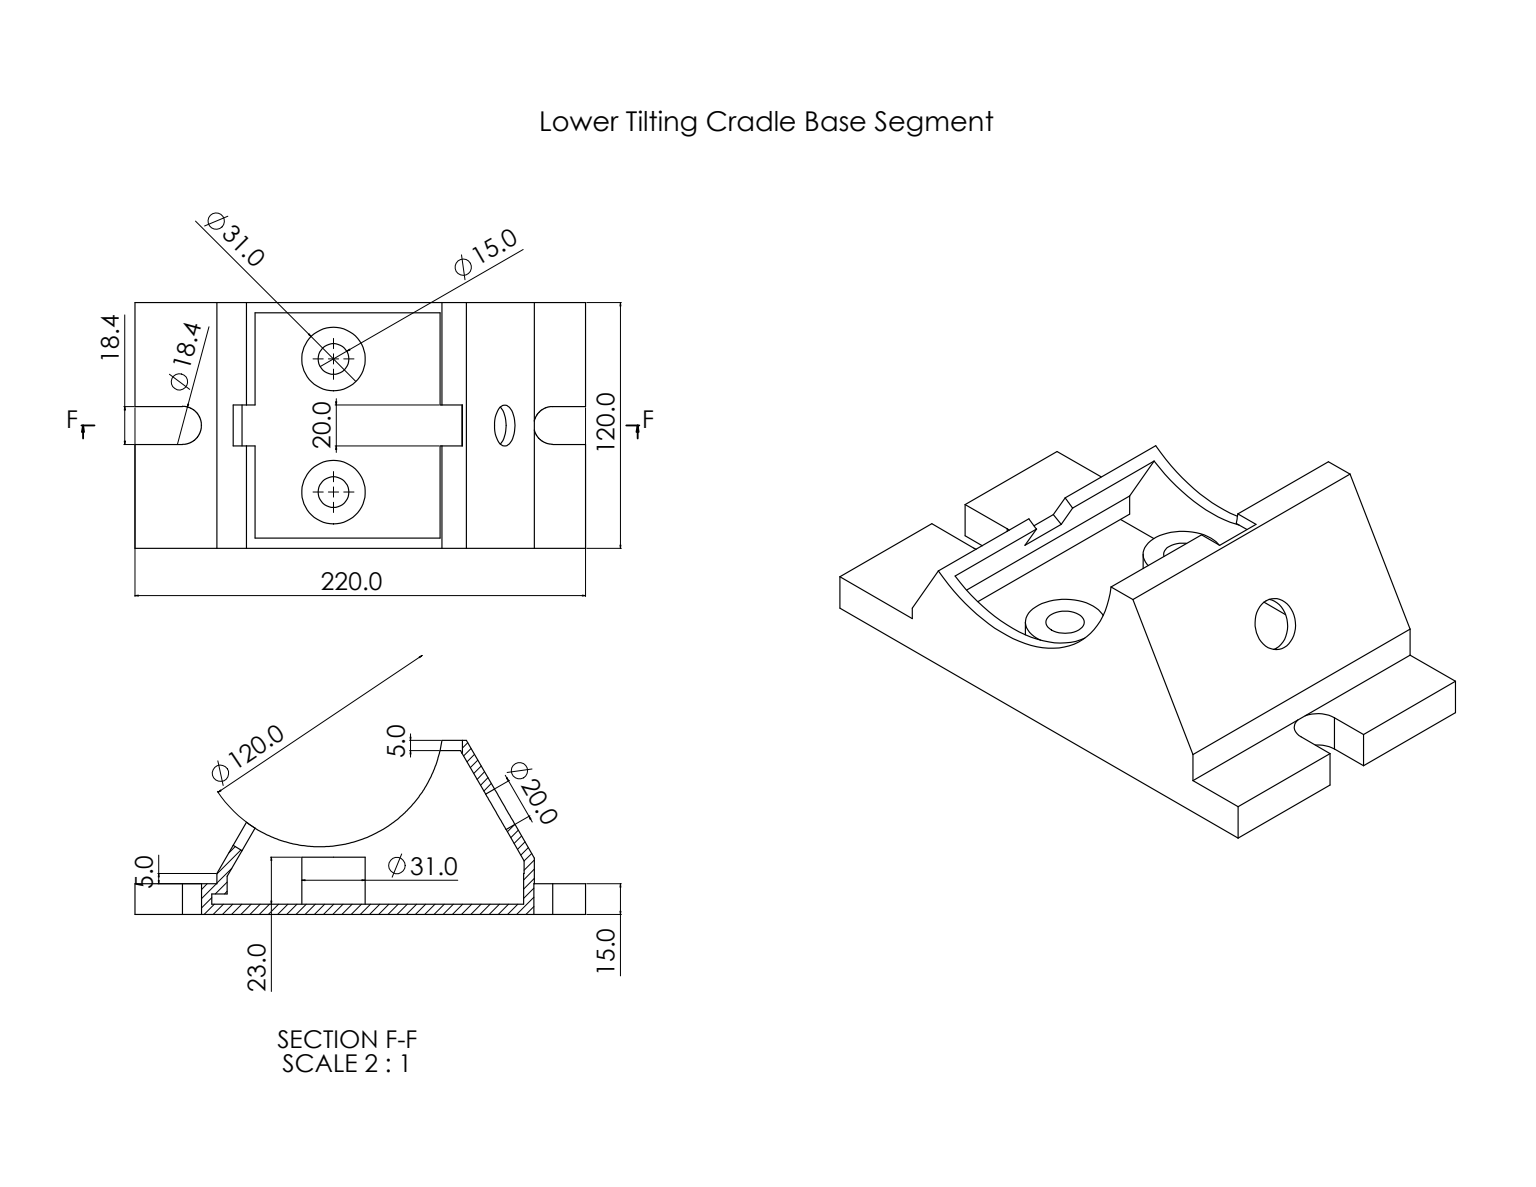
ISO-10303-21;
HEADER;
FILE_DESCRIPTION (('STEP AP214'),
    '1' );
FILE_NAME ('Lower Tilting Cradle Base Segment.step',
    '2026-10-24T22:31:37',
    ( '' ),
    ( '' ),
    'SwSTEP 2.0',
    'SolidWorks 2025',
    '' );
FILE_SCHEMA (( 'AUTOMOTIVE_DESIGN' ));
ENDSEC;

DATA;
#96=ADVANCED_FACE ( 'NONE', ( #87601 ), #64731, .F. ) ;
#141=ORIENTED_EDGE ( 'NONE', *, *, #32045, .F. ) ;
#200=ORIENTED_EDGE ( 'NONE', *, *, #33555, .T. ) ;
#230=LINE ( 'NONE', #68626, #5643 ) ;
#306=EDGE_CURVE ( 'NONE', #13446, #76018, #73820, .T. ) ;
#355=EDGE_CURVE ( 'NONE', #21265, #77716, #63095, .T. ) ;
#362=LINE ( 'NONE', #55534, #72254 ) ;
#380=DIRECTION ( 'NONE',  ( 0.000000000000000000, 1.000000000000000000, 0.000000000000000000 ) ) ;
#391=DIRECTION ( 'NONE',  ( 0.000000000000000000, 0.000000000000000000, 1.000000000000000000 ) ) ;
#453=CARTESIAN_POINT ( 'NONE',  ( -13.11024591527723437, 27.99999999999999645, -17.00000000000016698 ) ) ;
#496=ORIENTED_EDGE ( 'NONE', *, *, #84432, .T. ) ;
#512=DIRECTION ( 'NONE',  ( -1.000000000000000000, 0.000000000000000000, 5.984665299743594308E-16 ) ) ;
#589=ORIENTED_EDGE ( 'NONE', *, *, #57818, .F. ) ;
#618=PLANE ( 'NONE',  #9162 ) ;
#695=DIRECTION ( 'NONE',  ( 0.000000000000000000, 0.000000000000000000, 1.000000000000000000 ) ) ;
#707=ORIENTED_EDGE ( 'NONE', *, *, #77798, .F. ) ;
#714=CARTESIAN_POINT ( 'NONE',  ( -19.65312891409030271, 93.06504152958497400, -55.00000000000000000 ) ) ;
#795=EDGE_CURVE ( 'NONE', #82833, #80375, #31434, .T. ) ;
#809=CARTESIAN_POINT ( 'NONE',  ( 79.99999999999998579, 20.00000000000000000, 2.622423327744102917 ) ) ;
#830=LINE ( 'NONE', #47917, #18689 ) ;
#891=DIRECTION ( 'NONE',  ( 0.5000000000000014433, -0.8660254037844379305, 0.000000000000000000 ) ) ;
#949=VECTOR ( 'NONE', #67160, 1000.000000000000000 ) ;
#974=ORIENTED_EDGE ( 'NONE', *, *, #10004, .T. ) ;
#1001=EDGE_CURVE ( 'NONE', #40825, #22518, #21739, .T. ) ;
#1015=VECTOR ( 'NONE', #6214, 1000.000000000000227 ) ;
#1051=LINE ( 'NONE', #62833, #74374 ) ;
#1061=VECTOR ( 'NONE', #41991, 1000.000000000000000 ) ;
#1120=ORIENTED_EDGE ( 'NONE', *, *, #15724, .F. ) ;
#1321=CARTESIAN_POINT ( 'NONE',  ( -86.81108781737714253, 15.00000000000000000, -9.212605237762131694 ) ) ;
#1337=ORIENTED_EDGE ( 'NONE', *, *, #6609, .F. ) ;
#1350=AXIS2_PLACEMENT_3D ( 'NONE', #58082, #80942, #42854 ) ;
#1420=LINE ( 'NONE', #1917, #15890 ) ;
#1481=ORIENTED_EDGE ( 'NONE', *, *, #81998, .F. ) ;
#1496=EDGE_CURVE ( 'NONE', #63991, #3825, #52387, .T. ) ;
#1501=AXIS2_PLACEMENT_3D ( 'NONE', #64077, #39737, #47853 ) ;
#1530=VECTOR ( 'NONE', #96037, 1000.000000000000000 ) ;
#1591=VERTEX_POINT ( 'NONE', #34580 ) ;
#1615=DIRECTION ( 'NONE',  ( 0.000000000000000000, 0.000000000000000000, 1.000000000000000000 ) ) ;
#1638=EDGE_CURVE ( 'NONE', #76591, #63991, #42174, .T. ) ;
#1688=DIRECTION ( 'NONE',  ( 0.000000000000000000, 0.000000000000000000, 1.000000000000000000 ) ) ;
#1695=EDGE_LOOP ( 'NONE', ( #50576, #69212, #82002, #45259 ) ) ;
#1737=DIRECTION ( 'NONE',  ( -0.000000000000000000, -0.000000000000000000, -1.000000000000000000 ) ) ;
#1780=DIRECTION ( 'NONE',  ( 0.000000000000000000, 0.000000000000000000, -1.000000000000000000 ) ) ;
#1783=ORIENTED_EDGE ( 'NONE', *, *, #22842, .T. ) ;
#1815=ADVANCED_FACE ( 'NONE', ( #67970 ), #60345, .F. ) ;
#1828=ADVANCED_FACE ( 'NONE', ( #24857 ), #62342, .F. ) ;
#1839=ORIENTED_EDGE ( 'NONE', *, *, #94634, .T. ) ;
#1906=LINE ( 'NONE', #2413, #45145 ) ;
#1917=CARTESIAN_POINT ( 'NONE',  ( -86.81108781737714253, -8.000000000000000000, 9.212605237762131694 ) ) ;
#1932=DIRECTION ( 'NONE',  ( 0.000000000000000000, 0.000000000000000000, 1.000000000000000000 ) ) ;
#1982=CARTESIAN_POINT ( 'NONE',  ( -13.11024591527723437, 4.999999999999999112, -17.00000000000016698 ) ) ;
#2042=CARTESIAN_POINT ( 'NONE',  ( 84.99999999999998579, 14.99999999999999467, 59.99999999999999289 ) ) ;
#2063=LINE ( 'NONE', #94289, #52221 ) ;
#2065=CARTESIAN_POINT ( 'NONE',  ( -13.11024591527734628, 4.999999999999999112, 32.50000000000000000 ) ) ;
#2134=ORIENTED_EDGE ( 'NONE', *, *, #91860, .T. ) ;
#2145=DIRECTION ( 'NONE',  ( -0.000000000000000000, -0.000000000000000000, -1.000000000000000000 ) ) ;
#2176=DIRECTION ( 'NONE',  ( 0.000000000000000000, -1.000000000000000000, 0.000000000000000000 ) ) ;
#2190=EDGE_CURVE ( 'NONE', #32767, #65750, #49994, .T. ) ;
#2239=DIRECTION ( 'NONE',  ( 0.000000000000000000, 0.000000000000000000, 1.000000000000000000 ) ) ;
#2341=ORIENTED_EDGE ( 'NONE', *, *, #58740, .T. ) ;
#2347=CIRCLE ( 'NONE', #75171, 7.499999999999996447 ) ;
#2349=ORIENTED_EDGE ( 'NONE', *, *, #73320, .F. ) ;
#2360=ADVANCED_FACE ( 'NONE', ( #38759 ), #24562, .T. ) ;
#2399=CARTESIAN_POINT ( 'NONE',  ( -105.0000000000000000, 10.00000000000000000, 54.99999999999999289 ) ) ;
#2413=CARTESIAN_POINT ( 'NONE',  ( -110.0000000000000000, 0.000000000000000000, 59.99999999999999289 ) ) ;
#2480=DIRECTION ( 'NONE',  ( 0.8660254037844380415, -0.5000000000000011102, 0.000000000000000000 ) ) ;
#2502=( GEOMETRIC_REPRESENTATION_CONTEXT ( 3 ) GLOBAL_UNCERTAINTY_ASSIGNED_CONTEXT ( ( #47345 ) ) GLOBAL_UNIT_ASSIGNED_CONTEXT ( ( #60965, #8282, #62449 ) ) REPRESENTATION_CONTEXT ( 'NONE', 'WORKASPACE' ) );
#2516=DIRECTION ( 'NONE',  ( 1.000000000000000000, 1.830829162166278276E-15, -8.881784197001251337E-16 ) ) ;
#2552=AXIS2_PLACEMENT_3D ( 'NONE', #64991, #65977, #19896 ) ;
#2582=FACE_OUTER_BOUND ( 'NONE', #41311, .T. ) ;
#2594=DIRECTION ( 'NONE',  ( 0.000000000000000000, 0.000000000000000000, 1.000000000000000000 ) ) ;
#2612=AXIS2_PLACEMENT_3D ( 'NONE', #76038, #24793, #3035 ) ;
#2613=CARTESIAN_POINT ( 'NONE',  ( -105.0000000000000000, 9.999999999999998224, 59.99999999999999289 ) ) ;
#2619=VERTEX_POINT ( 'NONE', #58345 ) ;
#2655=DIRECTION ( 'NONE',  ( -0.000000000000000000, -0.000000000000000000, -1.000000000000000000 ) ) ;
#2678=DIRECTION ( 'NONE',  ( 0.000000000000000000, 0.000000000000000000, -1.000000000000000000 ) ) ;
#2723=CARTESIAN_POINT ( 'NONE',  ( -19.65312891409030271, 93.06504152958497400, 59.99999999999999289 ) ) ;
#2734=VERTEX_POINT ( 'NONE', #83185 ) ;
#2737=PLANE ( 'NONE',  #87118 ) ;
#2827=VERTEX_POINT ( 'NONE', #59838 ) ;
#2936=CIRCLE ( 'NONE', #87075, 60.00000000000002132 ) ;
#3035=DIRECTION ( 'NONE',  ( 0.000000000000000000, 0.000000000000000000, -1.000000000000000000 ) ) ;
#3071=CARTESIAN_POINT ( 'NONE',  ( 49.80235952159635815, 85.00000000000000000, -10.00000000000000000 ) ) ;
#3110=ORIENTED_EDGE ( 'NONE', *, *, #2190, .F. ) ;
#3139=DIRECTION ( 'NONE',  ( 1.000000000000000000, 0.000000000000000000, -5.984665299743594308E-16 ) ) ;
#3142=CARTESIAN_POINT ( 'NONE',  ( -62.06645187246650153, 33.74130844118091943, -10.00000000000000000 ) ) ;
#3148=ORIENTED_EDGE ( 'NONE', *, *, #31406, .T. ) ;
#3152=DIRECTION ( 'NONE',  ( 0.000000000000000000, 1.000000000000000000, 0.000000000000000000 ) ) ;
#3243=VERTEX_POINT ( 'NONE', #24231 ) ;
#3315=VECTOR ( 'NONE', #35069, 1000.000000000000000 ) ;
#3330=ADVANCED_FACE ( 'NONE', ( #55109 ), #48016, .T. ) ;
#3355=ORIENTED_EDGE ( 'NONE', *, *, #29773, .F. ) ;
#3356=ADVANCED_FACE ( 'NONE', ( #3449 ), #66230, .F. ) ;
#3421=LINE ( 'NONE', #24689, #27382 ) ;
#3432=CARTESIAN_POINT ( 'NONE',  ( -55.56624327025929944, 44.99999999999998579, 59.99999999999999289 ) ) ;
#3449=FACE_OUTER_BOUND ( 'NONE', #56451, .T. ) ;
#3521=CARTESIAN_POINT ( 'NONE',  ( 93.96857342517719758, 20.00000000000000000, 0.000000000000000000 ) ) ;
#3534=EDGE_CURVE ( 'NONE', #13682, #35306, #43152, .T. ) ;
#3654=ADVANCED_FACE ( 'NONE', ( #2582 ), #54741, .F. ) ;
#3712=PLANE ( 'NONE',  #92097 ) ;
#3743=LINE ( 'NONE', #65519, #77134 ) ;
#3763=PLANE ( 'NONE',  #69243 ) ;
#3799=CARTESIAN_POINT ( 'NONE',  ( -110.0000000000000142, 0.000000000000000000, -9.212605237762106825 ) ) ;
#3816=DIRECTION ( 'NONE',  ( 0.000000000000000000, 0.000000000000000000, -1.000000000000000000 ) ) ;
#3825=VERTEX_POINT ( 'NONE', #88221 ) ;
#3844=CARTESIAN_POINT ( 'NONE',  ( 93.96857342517718337, -8.000000000000000000, 9.212605237762133470 ) ) ;
#3867=ORIENTED_EDGE ( 'NONE', *, *, #82047, .F. ) ;
#3924=VECTOR ( 'NONE', #40267, 1000.000000000000000 ) ;
#3975=EDGE_CURVE ( 'NONE', #49412, #13462, #77466, .T. ) ;
#4096=DIRECTION ( 'NONE',  ( 0.000000000000000000, 1.000000000000000000, 0.000000000000000000 ) ) ;
#4152=DIRECTION ( 'NONE',  ( 0.000000000000000000, 0.000000000000000000, -1.000000000000000000 ) ) ;
#4184=ORIENTED_EDGE ( 'NONE', *, *, #66078, .F. ) ;
#4251=CARTESIAN_POINT ( 'NONE',  ( -110.0000000000000142, 15.00000000000000000, 9.212605237762145904 ) ) ;
#4359=ORIENTED_EDGE ( 'NONE', *, *, #28939, .T. ) ;
#4366=CYLINDRICAL_SURFACE ( 'NONE', #60771, 9.212605237762131694 ) ;
#4442=DIRECTION ( 'NONE',  ( 1.000000000000000000, 0.000000000000000000, -1.082076799516502080E-16 ) ) ;
#4463=CIRCLE ( 'NONE', #23895, 12.50000000000000000 ) ;
#4556=ORIENTED_EDGE ( 'NONE', *, *, #75424, .F. ) ;
#4573=EDGE_CURVE ( 'NONE', #69960, #75741, #26759, .T. ) ;
#4621=AXIS2_PLACEMENT_3D ( 'NONE', #87595, #71332, #80969 ) ;
#4634=DIRECTION ( 'NONE',  ( 0.000000000000000000, 0.000000000000000000, -1.000000000000000000 ) ) ;
#4646=VECTOR ( 'NONE', #2655, 1000.000000000000000 ) ;
#4703=DIRECTION ( 'NONE',  ( 1.000000000000000000, 0.000000000000000000, 0.000000000000000000 ) ) ;
#4729=DIRECTION ( 'NONE',  ( -0.8660254037844379305, -0.5000000000000014433, 0.000000000000000000 ) ) ;
#4851=ORIENTED_EDGE ( 'NONE', *, *, #47272, .F. ) ;
#4873=DIRECTION ( 'NONE',  ( -1.000000000000000000, -0.000000000000000000, 5.984665299743594308E-16 ) ) ;
#4874=DIRECTION ( 'NONE',  ( 0.000000000000000000, 1.000000000000000000, 0.000000000000000000 ) ) ;
#4903=DIRECTION ( 'NONE',  ( -0.5000000000000011102, -0.8660254037844380415, -0.000000000000000000 ) ) ;
#4960=PLANE ( 'NONE',  #88631 ) ;
#5118=AXIS2_PLACEMENT_3D ( 'NONE', #2065, #16250, #78065 ) ;
#5284=DIRECTION ( 'NONE',  ( 0.000000000000000000, 1.000000000000000000, 0.000000000000000000 ) ) ;
#5306=CARTESIAN_POINT ( 'NONE',  ( 84.99999999999998579, 14.99999999999999467, 59.99999999999999289 ) ) ;
#5595=CIRCLE ( 'NONE', #20150, 60.00000000000001421 ) ;
#5643=VECTOR ( 'NONE', #31115, 1000.000000000000114 ) ;
#5699=EDGE_LOOP ( 'NONE', ( #1337, #34998 ) ) ;
#5700=VERTEX_POINT ( 'NONE', #98265 ) ;
#5808=DIRECTION ( 'NONE',  ( -0.000000000000000000, -0.000000000000000000, -1.000000000000000000 ) ) ;
#5823=ORIENTED_EDGE ( 'NONE', *, *, #86339, .F. ) ;
#5827=LINE ( 'NONE', #3844, #18476 ) ;
#5837=ORIENTED_EDGE ( 'NONE', *, *, #81547, .T. ) ;
#5873=VECTOR ( 'NONE', #53819, 1000.000000000000000 ) ;
#5910=CIRCLE ( 'NONE', #22031, 15.50000000000000000 ) ;
#5942=ORIENTED_EDGE ( 'NONE', *, *, #40283, .T. ) ;
#5969=ORIENTED_EDGE ( 'NONE', *, *, #7524, .T. ) ;
#5970=ORIENTED_EDGE ( 'NONE', *, *, #29773, .T. ) ;
#5991=AXIS2_PLACEMENT_3D ( 'NONE', #32252, #79900, #41341 ) ;
#6026=EDGE_CURVE ( 'NONE', #2734, #60148, #55618, .T. ) ;
#6054=ORIENTED_EDGE ( 'NONE', *, *, #88067, .T. ) ;
#6070=LINE ( 'NONE', #52657, #28606 ) ;
#6085=VERTEX_POINT ( 'NONE', #73847 ) ;
#6136=CARTESIAN_POINT ( 'NONE',  ( -110.0000000000000000, 0.000000000000000000, 59.99999999999999289 ) ) ;
#6153=PLANE ( 'NONE',  #48095 ) ;
#6214=DIRECTION ( 'NONE',  ( 0.2237140788069379993, 0.9746548163034761680, 0.000000000000000000 ) ) ;
#6254=AXIS2_PLACEMENT_3D ( 'NONE', #24289, #15673, #54664 ) ;
#6269=AXIS2_PLACEMENT_3D ( 'NONE', #92824, #77613, #84732 ) ;
#6316=DIRECTION ( 'NONE',  ( 0.000000000000000000, 0.000000000000000000, 1.000000000000000000 ) ) ;
#6355=EDGE_LOOP ( 'NONE', ( #98084, #4556, #76845, #81766, #17453 ) ) ;
#6415=ORIENTED_EDGE ( 'NONE', *, *, #27524, .T. ) ;
#6596=ORIENTED_EDGE ( 'NONE', *, *, #1496, .F. ) ;
#6609=EDGE_CURVE ( 'NONE', #29494, #48939, #74160, .T. ) ;
#6622=FACE_BOUND ( 'NONE', #64006, .T. ) ;
#6637=ORIENTED_EDGE ( 'NONE', *, *, #81998, .T. ) ;
#6682=ORIENTED_EDGE ( 'NONE', *, *, #31600, .F. ) ;
#6715=DIRECTION ( 'NONE',  ( -0.5143720371616018472, -0.8575671445351807920, 0.000000000000000000 ) ) ;
#6739=LINE ( 'NONE', #52819, #73963 ) ;
#6802=DIRECTION ( 'NONE',  ( 0.000000000000000000, 1.000000000000000000, 0.000000000000000000 ) ) ;
#6809=AXIS2_PLACEMENT_3D ( 'NONE', #78960, #63728, #94664 ) ;
#6810=VERTEX_POINT ( 'NONE', #43237 ) ;
#6812=CARTESIAN_POINT ( 'NONE',  ( -13.11024591527723615, 6.000000000000000000, -32.50000000000017053 ) ) ;
#6816=VERTEX_POINT ( 'NONE', #4251 ) ;
#6907=EDGE_CURVE ( 'NONE', #63624, #98201, #37138, .T. ) ;
#6910=ORIENTED_EDGE ( 'NONE', *, *, #53077, .F. ) ;
#6958=ORIENTED_EDGE ( 'NONE', *, *, #24976, .T. ) ;
#7024=AXIS2_PLACEMENT_3D ( 'NONE', #71217, #85967, #47876 ) ;
#7029=ADVANCED_FACE ( 'NONE', ( #63442 ), #31032, .F. ) ;
#7183=FACE_OUTER_BOUND ( 'NONE', #37313, .T. ) ;
#7187=EDGE_CURVE ( 'NONE', #44016, #33601, #45047, .T. ) ;
#7207=EDGE_CURVE ( 'NONE', #17355, #2827, #70957, .T. ) ;
#7210=LINE ( 'NONE', #84757, #83975 ) ;
#7221=LINE ( 'NONE', #23414, #59978 ) ;
#7346=CARTESIAN_POINT ( 'NONE',  ( -70.00000000000000000, 15.00000000000000000, 59.99999999999999289 ) ) ;
#7350=DIRECTION ( 'NONE',  ( -1.000000000000000000, -1.156482317317871331E-15, 0.000000000000000000 ) ) ;
#7425=VERTEX_POINT ( 'NONE', #97617 ) ;
#7524=EDGE_CURVE ( 'NONE', #39339, #33343, #52976, .T. ) ;
#7554=DIRECTION ( 'NONE',  ( 1.156482317317871331E-15, -1.000000000000000000, 0.000000000000000000 ) ) ;
#7558=DIRECTION ( 'NONE',  ( 1.156482317317871331E-15, -1.000000000000000000, 0.000000000000000000 ) ) ;
#7659=CARTESIAN_POINT ( 'NONE',  ( 110.0000000000000000, 0.000000000000000000, 9.212605237762131694 ) ) ;
#7663=ADVANCED_FACE ( 'NONE', ( #75564 ), #6153, .F. ) ;
#7781=DIRECTION ( 'NONE',  ( 0.000000000000000000, 1.000000000000000000, 0.000000000000000000 ) ) ;
#7838=ORIENTED_EDGE ( 'NONE', *, *, #18191, .T. ) ;
#7906=CARTESIAN_POINT ( 'NONE',  ( -65.00000000000000000, 10.00000000000000178, 59.99999999999999289 ) ) ;
#7952=DIRECTION ( 'NONE',  ( -0.000000000000000000, -1.000000000000000000, -0.000000000000000000 ) ) ;
#7991=CARTESIAN_POINT ( 'NONE',  ( -110.0000000000000426, 4.999999999999999112, -14.21260523776211215 ) ) ;
#8004=DIRECTION ( 'NONE',  ( 0.000000000000000000, 1.000000000000000000, 0.000000000000000000 ) ) ;
#8186=PLANE ( 'NONE',  #31771 ) ;
#8194=ORIENTED_EDGE ( 'NONE', *, *, #47470, .F. ) ;
#8199=EDGE_LOOP ( 'NONE', ( #54144, #36257 ) ) ;
#8205=EDGE_LOOP ( 'NONE', ( #12958, #2341, #55389, #75767, #70838 ) ) ;
#8272=CARTESIAN_POINT ( 'NONE',  ( -13.11024591527734628, 6.000000000000000000, 32.50000000000000000 ) ) ;
#8282=( NAMED_UNIT ( * ) PLANE_ANGLE_UNIT ( ) SI_UNIT ( $, .RADIAN. ) );
#8369=DIRECTION ( 'NONE',  ( -0.000000000000000000, -1.000000000000000000, -0.000000000000000000 ) ) ;
#8388=ORIENTED_EDGE ( 'NONE', *, *, #78097, .T. ) ;
#8445=CARTESIAN_POINT ( 'NONE',  ( -86.81108781737714253, 0.000000000000000000, 9.212605237762135246 ) ) ;
#8589=EDGE_CURVE ( 'NONE', #53003, #57163, #80727, .T. ) ;
#8604=VERTEX_POINT ( 'NONE', #50754 ) ;
#8678=FACE_OUTER_BOUND ( 'NONE', #67367, .T. ) ;
#8699=VECTOR ( 'NONE', #97023, 1000.000000000000000 ) ;
#8731=CARTESIAN_POINT ( 'NONE',  ( -51.42721978966704910, 42.16899896210639298, 54.99999999999999289 ) ) ;
#8799=EDGE_CURVE ( 'NONE', #87128, #2619, #29184, .T. ) ;
#8808=ORIENTED_EDGE ( 'NONE', *, *, #31406, .F. ) ;
#8871=PLANE ( 'NONE',  #1501 ) ;
#8885=CARTESIAN_POINT ( 'NONE',  ( -13.11024591527734628, 27.99999999999999645, 25.00000000000000000 ) ) ;
#8915=ORIENTED_EDGE ( 'NONE', *, *, #13828, .T. ) ;
#8959=LINE ( 'NONE', #26170, #85362 ) ;
#9037=ORIENTED_EDGE ( 'NONE', *, *, #13828, .F. ) ;
#9079=CARTESIAN_POINT ( 'NONE',  ( -19.65312891409015350, 9.999999999999801048, 54.99999999999999289 ) ) ;
#9162=AXIS2_PLACEMENT_3D ( 'NONE', #95743, #57171, #49580 ) ;
#9173=VERTEX_POINT ( 'NONE', #42488 ) ;
#9320=VERTEX_POINT ( 'NONE', #20219 ) ;
#9368=ORIENTED_EDGE ( 'NONE', *, *, #75468, .T. ) ;
#9384=ORIENTED_EDGE ( 'NONE', *, *, #43885, .F. ) ;
#9432=EDGE_LOOP ( 'NONE', ( #66152, #28594, #66415, #75582, #49979, #14045, #77775, #974, #49654, #44163, #32256 ) ) ;
#9471=VECTOR ( 'NONE', #42394, 1000.000000000000000 ) ;
#9485=CARTESIAN_POINT ( 'NONE',  ( -105.0000000000000000, 4.999999999999999112, 59.99999999999999289 ) ) ;
#9546=AXIS2_PLACEMENT_3D ( 'NONE', #63378, #15764, #48176 ) ;
#9599=EDGE_CURVE ( 'NONE', #91585, #32767, #2936, .T. ) ;
#9722=VERTEX_POINT ( 'NONE', #3432 ) ;
#9799=CARTESIAN_POINT ( 'NONE',  ( 80.66987298107778770, 24.99999999999998579, 10.00000000000000178 ) ) ;
#9844=CARTESIAN_POINT ( 'NONE',  ( -13.11024591527734628, 6.000000000000000000, -32.50000000000000000 ) ) ;
#10004=EDGE_CURVE ( 'NONE', #64385, #49158, #36788, .T. ) ;
#10043=ORIENTED_EDGE ( 'NONE', *, *, #16457, .T. ) ;
#10074=EDGE_LOOP ( 'NONE', ( #30260, #11587, #30906, #80828 ) ) ;
#10076=DIRECTION ( 'NONE',  ( 1.000000000000000000, 0.000000000000000000, -5.984665299743594308E-16 ) ) ;
#10299=ORIENTED_EDGE ( 'NONE', *, *, #31863, .F. ) ;
#10312=EDGE_CURVE ( 'NONE', #48468, #65117, #65086, .T. ) ;
#10345=EDGE_LOOP ( 'NONE', ( #76741, #15276, #27131, #45942, #31110, #99138, #10299, #26392 ) ) ;
#10427=ORIENTED_EDGE ( 'NONE', *, *, #3975, .F. ) ;
#10437=ORIENTED_EDGE ( 'NONE', *, *, #100044, .T. ) ;
#10531=FACE_OUTER_BOUND ( 'NONE', #76117, .T. ) ;
#10552=DIRECTION ( 'NONE',  ( 0.000000000000000000, 1.000000000000000000, 0.000000000000000000 ) ) ;
#10581=ORIENTED_EDGE ( 'NONE', *, *, #84432, .F. ) ;
#10673=VERTEX_POINT ( 'NONE', #76675 ) ;
#10758=VECTOR ( 'NONE', #96320, 1000.000000000000000 ) ;
#10765=VECTOR ( 'NONE', #25144, 1000.000000000000000 ) ;
#10827=EDGE_LOOP ( 'NONE', ( #589, #87160 ) ) ;
#10831=CARTESIAN_POINT ( 'NONE',  ( -13.11024591527734451, 15.00000000000000000, 40.00000000000000000 ) ) ;
#10845=ORIENTED_EDGE ( 'NONE', *, *, #58080, .F. ) ;
#10860=CARTESIAN_POINT ( 'NONE',  ( -104.9999999999999858, 93.06504152958497400, 54.99999999999999289 ) ) ;
#10886=EDGE_CURVE ( 'NONE', #16870, #13446, #1051, .T. ) ;
#10992=CARTESIAN_POINT ( 'NONE',  ( -86.81108781737714253, -8.000000000000000000, 0.000000000000000000 ) ) ;
#11110=AXIS2_PLACEMENT_3D ( 'NONE', #69782, #8004, #391 ) ;
#11124=DIRECTION ( 'NONE',  ( 0.000000000000000000, 0.000000000000000000, 1.000000000000000000 ) ) ;
#11193=ORIENTED_EDGE ( 'NONE', *, *, #37375, .F. ) ;
#11352=CIRCLE ( 'NONE', #22592, 15.50000000000000000 ) ;
#11489=CARTESIAN_POINT ( 'NONE',  ( -110.0000000000000142, 15.00000000000000000, -9.212605237762117483 ) ) ;
#11554=CARTESIAN_POINT ( 'NONE',  ( 110.0000000000000000, 15.00000000000003908, 59.99999999999999289 ) ) ;
#11587=ORIENTED_EDGE ( 'NONE', *, *, #77834, .T. ) ;
#11634=CIRCLE ( 'NONE', #5118, 15.50000000000000000 ) ;
#11698=CARTESIAN_POINT ( 'NONE',  ( -51.42721978966704910, 42.16899896210637877, -10.00000000000000000 ) ) ;
#11761=EDGE_CURVE ( 'NONE', #48169, #49525, #24485, .T. ) ;
#11821=EDGE_LOOP ( 'NONE', ( #39278, #9037, #8808, #19989, #96576, #43587, #74254, #52410, #26033, #19655, #96496, #91414 ) ) ;
#11899=DIRECTION ( 'NONE',  ( 0.000000000000000000, 0.000000000000000000, 1.000000000000000000 ) ) ;
#11936=PLANE ( 'NONE',  #64222 ) ;
#11950=ORIENTED_EDGE ( 'NONE', *, *, #26764, .F. ) ;
#12007=ADVANCED_FACE ( 'NONE', ( #63863 ), #80613, .F. ) ;
#12029=PLANE ( 'NONE',  #28013 ) ;
#12083=ORIENTED_EDGE ( 'NONE', *, *, #36288, .F. ) ;
#12112=CARTESIAN_POINT ( 'NONE',  ( 110.0000000000000142, 15.00000000000000000, 1.387778780781445676E-14 ) ) ;
#12211=EDGE_CURVE ( 'NONE', #6816, #59735, #88555, .T. ) ;
#12313=CARTESIAN_POINT ( 'NONE',  ( 51.80235952159636525, 85.00000000000000000, 59.99999999999999289 ) ) ;
#12429=LINE ( 'NONE', #53394, #94437 ) ;
#12512=VECTOR ( 'NONE', #75516, 1000.000000000000000 ) ;
#12543=VERTEX_POINT ( 'NONE', #16466 ) ;
#12578=AXIS2_PLACEMENT_3D ( 'NONE', #99825, #37496, #29910 ) ;
#12666=ORIENTED_EDGE ( 'NONE', *, *, #98157, .T. ) ;
#12680=EDGE_LOOP ( 'NONE', ( #77334, #100033, #5823, #10437, #80569, #73665, #85880, #95077 ) ) ;
#12804=DIRECTION ( 'NONE',  ( -0.000000000000000000, -1.000000000000000000, -0.000000000000000000 ) ) ;
#12934=LINE ( 'NONE', #67598, #31996 ) ;
#12958=ORIENTED_EDGE ( 'NONE', *, *, #17895, .F. ) ;
#12959=DIRECTION ( 'NONE',  ( -0.000000000000000000, 1.000000000000000000, -0.000000000000000000 ) ) ;
#13009=AXIS2_PLACEMENT_3D ( 'NONE', #23110, #25707, #57079 ) ;
#13040=ORIENTED_EDGE ( 'NONE', *, *, #66674, .T. ) ;
#13072=DIRECTION ( 'NONE',  ( -1.000000000000000000, 0.000000000000000000, 0.000000000000000000 ) ) ;
#13090=CARTESIAN_POINT ( 'NONE',  ( 79.99999999999998579, 14.99999999999998934, 59.99999999999999289 ) ) ;
#13110=CARTESIAN_POINT ( 'NONE',  ( -19.65312891409030271, 93.06504152958497400, -59.99999999999999289 ) ) ;
#13122=LINE ( 'NONE', #59688, #54631 ) ;
#13180=CARTESIAN_POINT ( 'NONE',  ( 38.90713653809340400, 79.99999999999998579, 54.99999999999999289 ) ) ;
#13291=VERTEX_POINT ( 'NONE', #46213 ) ;
#13311=DIRECTION ( 'NONE',  ( 0.8660254037844378194, 0.5000000000000015543, -0.000000000000000000 ) ) ;
#13402=ORIENTED_EDGE ( 'NONE', *, *, #64126, .F. ) ;
#13446=VERTEX_POINT ( 'NONE', #75534 ) ;
#13462=VERTEX_POINT ( 'NONE', #92749 ) ;
#13538=ORIENTED_EDGE ( 'NONE', *, *, #68927, .F. ) ;
#13545=EDGE_LOOP ( 'NONE', ( #63281, #18529, #82853, #24110 ) ) ;
#13556=DIRECTION ( 'NONE',  ( 1.235257323912246174E-15, 1.000000000000000000, -0.000000000000000000 ) ) ;
#13666=EDGE_LOOP ( 'NONE', ( #10427, #25237, #37357, #83611 ) ) ;
#13682=VERTEX_POINT ( 'NONE', #21114 ) ;
#13701=VECTOR ( 'NONE', #25855, 1000.000000000000000 ) ;
#13798=CARTESIAN_POINT ( 'NONE',  ( -13.11024591527723615, 27.99999999999999645, -32.50000000000017053 ) ) ;
#13828=EDGE_CURVE ( 'NONE', #42192, #32489, #30686, .T. ) ;
#13842=DIRECTION ( 'NONE',  ( 0.000000000000000000, 0.000000000000000000, -1.000000000000000000 ) ) ;
#13904=DIRECTION ( 'NONE',  ( 0.000000000000000000, -0.000000000000000000, 1.000000000000000000 ) ) ;
#13938=ORIENTED_EDGE ( 'NONE', *, *, #90752, .T. ) ;
#14045=ORIENTED_EDGE ( 'NONE', *, *, #6907, .T. ) ;
#14206=CARTESIAN_POINT ( 'NONE',  ( 84.99999999999998579, 14.99999999999999467, 59.99999999999999289 ) ) ;
#14229=DIRECTION ( 'NONE',  ( -0.000000000000000000, -0.000000000000000000, -1.000000000000000000 ) ) ;
#14282=CARTESIAN_POINT ( 'NONE',  ( -86.81108781737714253, 15.00000000000000000, 0.000000000000000000 ) ) ;
#14340=AXIS2_PLACEMENT_3D ( 'NONE', #98095, #81925, #21582 ) ;
#14428=VERTEX_POINT ( 'NONE', #91536 ) ;
#14468=ORIENTED_EDGE ( 'NONE', *, *, #70209, .F. ) ;
#14485=DIRECTION ( 'NONE',  ( -0.000000000000000000, -0.000000000000000000, -1.000000000000000000 ) ) ;
#14508=CARTESIAN_POINT ( 'NONE',  ( -13.11024591527734628, 27.99999999999999645, 32.50000000000000000 ) ) ;
#14525=EDGE_CURVE ( 'NONE', #65117, #18962, #26434, .T. ) ;
#14793=AXIS2_PLACEMENT_3D ( 'NONE', #45049, #21754, #60727 ) ;
#14802=CARTESIAN_POINT ( 'NONE',  ( -62.06645187246645889, 33.74130844118090522, -10.00000000000000000 ) ) ;
#14942=CARTESIAN_POINT ( 'NONE',  ( 51.80235952159637236, 80.00000000000000000, 10.00000000000000178 ) ) ;
#14978=AXIS2_PLACEMENT_3D ( 'NONE', #47021, #55597, #1932 ) ;
#14997=ADVANCED_BREP_SHAPE_REPRESENTATION ( '', ( #46005, #68784 ), #2502 ) ;
#15010=EDGE_CURVE ( 'NONE', #75521, #61222, #64605, .T. ) ;
#15036=ORIENTED_EDGE ( 'NONE', *, *, #73888, .T. ) ;
#15177=AXIS2_PLACEMENT_3D ( 'NONE', #21755, #36953, #83098 ) ;
#15179=ORIENTED_EDGE ( 'NONE', *, *, #91860, .F. ) ;
#15244=DIRECTION ( 'NONE',  ( 0.2237140788069379993, 0.9746548163034761680, 0.000000000000000000 ) ) ;
#15276=ORIENTED_EDGE ( 'NONE', *, *, #18587, .T. ) ;
#15305=DIRECTION ( 'NONE',  ( -0.5000000000000011102, -0.8660254037844380415, 0.000000000000000000 ) ) ;
#15350=CARTESIAN_POINT ( 'NONE',  ( 105.0000000000000000, 4.999999999999999112, -14.21260523776213347 ) ) ;
#15354=CARTESIAN_POINT ( 'NONE',  ( 0.000000000000000000, 0.000000000000000000, 0.000000000000000000 ) ) ;
#15356=FACE_BOUND ( 'NONE', #47426, .T. ) ;
#15381=ORIENTED_EDGE ( 'NONE', *, *, #74236, .T. ) ;
#15479=ORIENTED_EDGE ( 'NONE', *, *, #91225, .T. ) ;
#15497=LINE ( 'NONE', #55005, #80738 ) ;
#15629=EDGE_CURVE ( 'NONE', #57163, #35859, #66195, .T. ) ;
#15638=DIRECTION ( 'NONE',  ( 0.000000000000000000, -0.000000000000000000, -1.000000000000000000 ) ) ;
#15645=DIRECTION ( 'NONE',  ( 1.000000000000000000, 1.156482317317871331E-15, 0.000000000000000000 ) ) ;
#15650=DIRECTION ( 'NONE',  ( 0.000000000000000000, 0.000000000000000000, -1.000000000000000000 ) ) ;
#15673=DIRECTION ( 'NONE',  ( -1.000000000000000000, 0.000000000000000000, 0.000000000000000000 ) ) ;
#15716=VECTOR ( 'NONE', #66689, 1000.000000000000000 ) ;
#15724=EDGE_CURVE ( 'NONE', #54703, #17355, #72201, .T. ) ;
#15756=ADVANCED_FACE ( 'NONE', ( #42259 ), #57461, .F. ) ;
#15764=DIRECTION ( 'NONE',  ( -0.000000000000000000, -1.000000000000000000, -0.000000000000000000 ) ) ;
#15835=ORIENTED_EDGE ( 'NONE', *, *, #37375, .T. ) ;
#15890=VECTOR ( 'NONE', #54085, 1000.000000000000000 ) ;
#15966=CARTESIAN_POINT ( 'NONE',  ( -110.0000000000000426, 0.000000000000000000, -9.212605237762121035 ) ) ;
#16047=EDGE_CURVE ( 'NONE', #32489, #43945, #22719, .T. ) ;
#16057=DIRECTION ( 'NONE',  ( -1.000000000000000000, -1.156482317317871331E-15, 0.000000000000000000 ) ) ;
#16089=VECTOR ( 'NONE', #45606, 1000.000000000000000 ) ;
#16136=ORIENTED_EDGE ( 'NONE', *, *, #22842, .F. ) ;
#16152=CARTESIAN_POINT ( 'NONE',  ( -86.81108781737714253, 0.000000000000000000, -9.212605237762131694 ) ) ;
#16208=PLANE ( 'NONE',  #74040 ) ;
#16250=DIRECTION ( 'NONE',  ( 0.000000000000000000, 1.000000000000000000, 0.000000000000000000 ) ) ;
#16272=DIRECTION ( 'NONE',  ( 1.804112415015878984E-15, -1.000000000000000000, 0.000000000000000000 ) ) ;
#16419=FACE_OUTER_BOUND ( 'NONE', #56705, .T. ) ;
#16428=ADVANCED_FACE ( 'NONE', ( #57986 ), #88968, .F. ) ;
#16447=ORIENTED_EDGE ( 'NONE', *, *, #20153, .F. ) ;
#16457=EDGE_CURVE ( 'NONE', #61410, #77081, #63587, .T. ) ;
#16466=CARTESIAN_POINT ( 'NONE',  ( 38.90713653809340400, 79.99999999999998579, -10.00000000000000000 ) ) ;
#16556=ADVANCED_FACE ( 'NONE', ( #77171 ), #53850, .F. ) ;
#16631=VERTEX_POINT ( 'NONE', #15350 ) ;
#16669=DIRECTION ( 'NONE',  ( 1.000000000000000000, 0.000000000000000000, 0.000000000000000000 ) ) ;
#16684=CARTESIAN_POINT ( 'NONE',  ( 26.11609497015385983, 119.4899152597536869, -54.99999999999999289 ) ) ;
#16743=EDGE_CURVE ( 'NONE', #9173, #30330, #24735, .T. ) ;
#16769=DIRECTION ( 'NONE',  ( 0.000000000000000000, 0.000000000000000000, -1.000000000000000000 ) ) ;
#16792=VECTOR ( 'NONE', #27204, 1000.000000000000000 ) ;
#16834=CARTESIAN_POINT ( 'NONE',  ( 105.0000000000000000, 10.00000000000003197, 14.21260523776213347 ) ) ;
#16854=EDGE_LOOP ( 'NONE', ( #33876, #12083, #6958, #73122 ) ) ;
#16870=VERTEX_POINT ( 'NONE', #40358 ) ;
#16943=ORIENTED_EDGE ( 'NONE', *, *, #78097, .F. ) ;
#16986=ORIENTED_EDGE ( 'NONE', *, *, #60227, .F. ) ;
#16989=CARTESIAN_POINT ( 'NONE',  ( -13.11024591527734451, 4.999999999999999112, 48.00000000000000000 ) ) ;
#17032=FACE_OUTER_BOUND ( 'NONE', #28394, .T. ) ;
#17039=VECTOR ( 'NONE', #94840, 1000.000000000000000 ) ;
#17142=DIRECTION ( 'NONE',  ( 0.000000000000000000, 1.000000000000000000, 0.000000000000000000 ) ) ;
#17165=EDGE_CURVE ( 'NONE', #13291, #77081, #84397, .T. ) ;
#17199=VERTEX_POINT ( 'NONE', #31138 ) ;
#17251=VERTEX_POINT ( 'NONE', #67037 ) ;
#17260=VECTOR ( 'NONE', #40711, 1000.000000000000000 ) ;
#17276=DIRECTION ( 'NONE',  ( -0.000000000000000000, 0.000000000000000000, -1.000000000000000000 ) ) ;
#17337=VECTOR ( 'NONE', #86046, 1000.000000000000000 ) ;
#17353=DIRECTION ( 'NONE',  ( 0.000000000000000000, 0.000000000000000000, -1.000000000000000000 ) ) ;
#17355=VERTEX_POINT ( 'NONE', #36631 ) ;
#17372=ORIENTED_EDGE ( 'NONE', *, *, #18775, .F. ) ;
#17453=ORIENTED_EDGE ( 'NONE', *, *, #78170, .T. ) ;
#17460=CARTESIAN_POINT ( 'NONE',  ( -13.11024591527734628, 15.00000000000000000, 32.50000000000000000 ) ) ;
#17463=CIRCLE ( 'NONE', #99987, 15.50000000000000000 ) ;
#17688=ORIENTED_EDGE ( 'NONE', *, *, #43573, .F. ) ;
#17758=ORIENTED_EDGE ( 'NONE', *, *, #50742, .F. ) ;
#17889=CARTESIAN_POINT ( 'NONE',  ( 93.96857342517719758, -8.000000000000000000, 0.000000000000000000 ) ) ;
#17895=EDGE_CURVE ( 'NONE', #61222, #49297, #66309, .T. ) ;
#17930=DIRECTION ( 'NONE',  ( 1.000000000000000000, -1.235257323912246174E-15, 0.000000000000000000 ) ) ;
#17975=PRODUCT_DEFINITION_CONTEXT ( 'detailed design', #31646, 'design' ) ;
#18100=LINE ( 'NONE', #41379, #46965 ) ;
#18127=DIRECTION ( 'NONE',  ( -0.000000000000000000, -1.000000000000000000, -0.000000000000000000 ) ) ;
#18136=DIRECTION ( 'NONE',  ( 0.000000000000000000, 0.000000000000000000, -1.000000000000000000 ) ) ;
#18191=EDGE_CURVE ( 'NONE', #98201, #61436, #31536, .T. ) ;
#18345=CIRCLE ( 'NONE', #57146, 14.21260523776213347 ) ;
#18390=LINE ( 'NONE', #48285, #93665 ) ;
#18431=ORIENTED_EDGE ( 'NONE', *, *, #28789, .F. ) ;
#18476=VECTOR ( 'NONE', #12959, 1000.000000000000000 ) ;
#18521=EDGE_CURVE ( 'NONE', #31869, #36246, #72575, .T. ) ;
#18529=ORIENTED_EDGE ( 'NONE', *, *, #83832, .T. ) ;
#18587=EDGE_CURVE ( 'NONE', #20674, #98683, #88813, .T. ) ;
#18623=VECTOR ( 'NONE', #73097, 999.9999999999998863 ) ;
#18666=ORIENTED_EDGE ( 'NONE', *, *, #18971, .T. ) ;
#18689=VECTOR ( 'NONE', #41316, 1000.000000000000000 ) ;
#18775=EDGE_CURVE ( 'NONE', #47896, #88729, #58018, .T. ) ;
#18893=LINE ( 'NONE', #9799, #18623 ) ;
#18904=EDGE_CURVE ( 'NONE', #7425, #52455, #74047, .T. ) ;
#18906=ORIENTED_EDGE ( 'NONE', *, *, #6026, .T. ) ;
#18962=VERTEX_POINT ( 'NONE', #97358 ) ;
#18965=LINE ( 'NONE', #73165, #88930 ) ;
#18971=EDGE_CURVE ( 'NONE', #9320, #94434, #27924, .T. ) ;
#18979=CIRCLE ( 'NONE', #31876, 12.50000000000000000 ) ;
#19001=DIRECTION ( 'NONE',  ( 0.000000000000000000, -1.000000000000000000, 0.000000000000000000 ) ) ;
#19017=EDGE_CURVE ( 'NONE', #76847, #17199, #59812, .T. ) ;
#19048=CARTESIAN_POINT ( 'NONE',  ( 93.96857342517719758, -8.000000000000000000, 0.000000000000000000 ) ) ;
#19056=ORIENTED_EDGE ( 'NONE', *, *, #7187, .T. ) ;
#19107=EDGE_CURVE ( 'NONE', #12543, #82272, #29425, .T. ) ;
#19121=CARTESIAN_POINT ( 'NONE',  ( -110.0000000000000142, 15.00000000000000000, 9.212605237762145904 ) ) ;
#19163=ORIENTED_EDGE ( 'NONE', *, *, #77798, .T. ) ;
#19219=ORIENTED_EDGE ( 'NONE', *, *, #75468, .F. ) ;
#19306=CIRCLE ( 'NONE', #75919, 7.500000000000000000 ) ;
#19321=CARTESIAN_POINT ( 'NONE',  ( -110.0000000000000142, 0.000000000000000000, -9.212605237762117483 ) ) ;
#19329=VECTOR ( 'NONE', #13311, 1000.000000000000000 ) ;
#19351=FACE_BOUND ( 'NONE', #10827, .T. ) ;
#19523=CARTESIAN_POINT ( 'NONE',  ( 110.0000000000000000, 15.00000000000003908, 59.99999999999999289 ) ) ;
#19655=ORIENTED_EDGE ( 'NONE', *, *, #15629, .F. ) ;
#19688=DIRECTION ( 'NONE',  ( 0.000000000000000000, 0.000000000000000000, 1.000000000000000000 ) ) ;
#19845=AXIS2_PLACEMENT_3D ( 'NONE', #38551, #92795, #47152 ) ;
#19896=DIRECTION ( 'NONE',  ( 1.110223024625156343E-15, -1.000000000000000000, 0.000000000000000000 ) ) ;
#19989=ORIENTED_EDGE ( 'NONE', *, *, #28077, .T. ) ;
#20018=LINE ( 'NONE', #45643, #35487 ) ;
#20150=AXIS2_PLACEMENT_3D ( 'NONE', #33625, #1737, #65021 ) ;
#20153=EDGE_CURVE ( 'NONE', #31618, #54703, #42384, .T. ) ;
#20169=CARTESIAN_POINT ( 'NONE',  ( 110.0000000000000000, 15.00000000000000000, 9.212605237762131694 ) ) ;
#20172=DIRECTION ( 'NONE',  ( -0.000000000000000000, 1.000000000000000000, -0.000000000000000000 ) ) ;
#20219=CARTESIAN_POINT ( 'NONE',  ( 49.65150239490934325, 78.72539382324355017, -10.00000000000000178 ) ) ;
#20236=CARTESIAN_POINT ( 'NONE',  ( 48.91560817564824504, 80.00000000000000000, 59.99999999999999289 ) ) ;
#20288=ORIENTED_EDGE ( 'NONE', *, *, #89441, .F. ) ;
#20316=( LENGTH_UNIT ( ) NAMED_UNIT ( * ) SI_UNIT ( .MILLI., .METRE. ) );
#20335=CARTESIAN_POINT ( 'NONE',  ( 79.99999999999998579, 9.999999999999985789, -2.622423327744149102 ) ) ;
#20515=CARTESIAN_POINT ( 'NONE',  ( -13.11024591527734628, 6.000000000000000000, 32.50000000000000000 ) ) ;
#20552=EDGE_CURVE ( 'NONE', #41822, #12543, #28399, .T. ) ;
#20639=DIRECTION ( 'NONE',  ( -0.8660254037844378194, -0.5000000000000014433, 0.000000000000000000 ) ) ;
#20674=VERTEX_POINT ( 'NONE', #43333 ) ;
#20681=FACE_OUTER_BOUND ( 'NONE', #49213, .T. ) ;
#20685=LINE ( 'NONE', #74893, #46224 ) ;
#20689=CARTESIAN_POINT ( 'NONE',  ( 49.80235952159635815, 85.00000000000000000, 10.00000000000000000 ) ) ;
#20781=DIRECTION ( 'NONE',  ( 0.000000000000000000, -1.000000000000000000, 0.000000000000000000 ) ) ;
#20796=ORIENTED_EDGE ( 'NONE', *, *, #85697, .F. ) ;
#20806=DIRECTION ( 'NONE',  ( 0.000000000000000000, 0.000000000000000000, -1.000000000000000000 ) ) ;
#20974=DIRECTION ( 'NONE',  ( -0.000000000000000000, -0.000000000000000000, -1.000000000000000000 ) ) ;
#20976=LINE ( 'NONE', #27575, #91869 ) ;
#21032=FACE_OUTER_BOUND ( 'NONE', #94666, .T. ) ;
#21114=CARTESIAN_POINT ( 'NONE',  ( -110.0000000000000000, 15.00000000000000000, -59.99999999999999289 ) ) ;
#21265=VERTEX_POINT ( 'NONE', #20689 ) ;
#21314=AXIS2_PLACEMENT_3D ( 'NONE', #48150, #79093, #85715 ) ;
#21345=LINE ( 'NONE', #6136, #62537 ) ;
#21391=CARTESIAN_POINT ( 'NONE',  ( 23.52134341065870160, 13.98415679381821342, 1.224646799147354045E-15 ) ) ;
#21408=DIRECTION ( 'NONE',  ( -0.000000000000000000, -1.000000000000000000, -0.000000000000000000 ) ) ;
#21422=CARTESIAN_POINT ( 'NONE',  ( -62.10935938174410609, 33.76704452855005201, -10.00000000000000000 ) ) ;
#21502=CARTESIAN_POINT ( 'NONE',  ( 70.48286763772495078, 52.64441083166268243, 0.000000000000000000 ) ) ;
#21521=ORIENTED_EDGE ( 'NONE', *, *, #50546, .F. ) ;
#21582=DIRECTION ( 'NONE',  ( 0.000000000000000000, 0.000000000000000000, -1.000000000000000000 ) ) ;
#21698=DIRECTION ( 'NONE',  ( 0.000000000000000000, 0.000000000000000000, 1.000000000000000000 ) ) ;
#21709=ADVANCED_FACE ( 'NONE', ( #73777 ), #4366, .F. ) ;
#21739=LINE ( 'NONE', #97764, #76463 ) ;
#21751=DIRECTION ( 'NONE',  ( -0.000000000000000000, -0.000000000000000000, -1.000000000000000000 ) ) ;
#21754=DIRECTION ( 'NONE',  ( 0.000000000000000000, 1.000000000000000000, 0.000000000000000000 ) ) ;
#21755=CARTESIAN_POINT ( 'NONE',  ( -86.81108781737714253, 4.999999999999999112, 0.000000000000000000 ) ) ;
#21787=EDGE_CURVE ( 'NONE', #52455, #57758, #60534, .T. ) ;
#21852=AXIS2_PLACEMENT_3D ( 'NONE', #9844, #40704, #2239 ) ;
#21884=LINE ( 'NONE', #90345, #31593 ) ;
#21942=CARTESIAN_POINT ( 'NONE',  ( 51.80235952159636525, 85.00000000000000000, 59.99999999999999289 ) ) ;
#21965=ORIENTED_EDGE ( 'NONE', *, *, #50546, .T. ) ;
#22031=AXIS2_PLACEMENT_3D ( 'NONE', #94095, #86021, #40829 ) ;
#22075=ADVANCED_FACE ( 'NONE', ( #70397 ), #45104, .F. ) ;
#22091=CARTESIAN_POINT ( 'NONE',  ( 84.99999999999997158, 27.49999999999999645, 59.99999999999999289 ) ) ;
#22174=VECTOR ( 'NONE', #88758, 1000.000000000000000 ) ;
#22238=VECTOR ( 'NONE', #92614, 1000.000000000000000 ) ;
#22268=CARTESIAN_POINT ( 'NONE',  ( -105.0000000000000000, -8.000000000000000000, 14.21260523776214235 ) ) ;
#22287=EDGE_CURVE ( 'NONE', #37352, #61117, #68778, .T. ) ;
#22291=( NAMED_UNIT ( * ) SI_UNIT ( $, .STERADIAN. ) SOLID_ANGLE_UNIT ( ) );
#22382=VECTOR ( 'NONE', #2145, 1000.000000000000000 ) ;
#22396=ORIENTED_EDGE ( 'NONE', *, *, #52325, .T. ) ;
#22490=DIRECTION ( 'NONE',  ( 0.000000000000000000, -0.000000000000000000, -1.000000000000000000 ) ) ;
#22518=VERTEX_POINT ( 'NONE', #78359 ) ;
#22575=DIRECTION ( 'NONE',  ( -1.000000000000000000, 0.000000000000000000, 5.984665299743594308E-16 ) ) ;
#22585=VERTEX_POINT ( 'NONE', #8445 ) ;
#22592=AXIS2_PLACEMENT_3D ( 'NONE', #41833, #74270, #72267 ) ;
#22631=AXIS2_PLACEMENT_3D ( 'NONE', #25362, #25887, #41553 ) ;
#22702=EDGE_CURVE ( 'NONE', #40435, #31854, #42813, .T. ) ;
#22719=LINE ( 'NONE', #100230, #58699 ) ;
#22739=EDGE_LOOP ( 'NONE', ( #48710, #69821, #6910, #66880 ) ) ;
#22777=ORIENTED_EDGE ( 'NONE', *, *, #54639, .F. ) ;
#22842=EDGE_CURVE ( 'NONE', #82272, #97333, #99717, .T. ) ;
#23062=CARTESIAN_POINT ( 'NONE',  ( -110.0000000000000284, 4.999999999999999112, 14.21260523776214590 ) ) ;
#23110=CARTESIAN_POINT ( 'NONE',  ( 93.96857342517719758, 15.00000000000000000, 0.000000000000000000 ) ) ;
#23207=EDGE_CURVE ( 'NONE', #38156, #22585, #48199, .T. ) ;
#23269=LINE ( 'NONE', #16684, #79125 ) ;
#23275=DIRECTION ( 'NONE',  ( -0.000000000000000000, -0.000000000000000000, -1.000000000000000000 ) ) ;
#23296=CARTESIAN_POINT ( 'NONE',  ( -13.11024591527734628, 6.000000000000000000, -32.50000000000000000 ) ) ;
#23338=SHAPE_DEFINITION_REPRESENTATION ( #28168, #35972 ) ;
#23361=DIRECTION ( 'NONE',  ( 1.000000000000000000, 1.804112415015878984E-15, 0.000000000000000000 ) ) ;
#23362=EDGE_CURVE ( 'NONE', #13462, #82272, #362, .T. ) ;
#23414=CARTESIAN_POINT ( 'NONE',  ( 39.80235952159635815, 84.99999999999998579, 59.99999999999999289 ) ) ;
#23415=CARTESIAN_POINT ( 'NONE',  ( 79.99999999999998579, 9.999999999999985789, -2.622423327744149102 ) ) ;
#23423=CARTESIAN_POINT ( 'NONE',  ( 110.0000000000000000, 0.000000000000000000, 59.99999999999999289 ) ) ;
#23457=DIRECTION ( 'NONE',  ( 1.000000000000000000, 0.000000000000000000, 0.000000000000000000 ) ) ;
#23507=CARTESIAN_POINT ( 'NONE',  ( -70.00000000000000000, 15.00000000000000000, 59.99999999999999289 ) ) ;
#23617=CARTESIAN_POINT ( 'NONE',  ( -57.77801984846012573, 31.16909059156539996, 10.00000000000000178 ) ) ;
#23767=CIRCLE ( 'NONE', #36717, 60.00000000000001421 ) ;
#23781=CARTESIAN_POINT ( 'NONE',  ( -70.00000000000000000, 15.00000000000000000, 59.99999999999999289 ) ) ;
#23895=AXIS2_PLACEMENT_3D ( 'NONE', #23296, #62286, #46592 ) ;
#23989=DIRECTION ( 'NONE',  ( 0.000000000000000000, 0.000000000000000000, 1.000000000000000000 ) ) ;
#24110=ORIENTED_EDGE ( 'NONE', *, *, #3534, .T. ) ;
#24231=CARTESIAN_POINT ( 'NONE',  ( -65.00000000000000000, 10.00000000000000000, -54.99999999999999289 ) ) ;
#24233=ORIENTED_EDGE ( 'NONE', *, *, #40702, .T. ) ;
#24277=DIRECTION ( 'NONE',  ( -0.000000000000000000, -0.000000000000000000, -1.000000000000000000 ) ) ;
#24289=CARTESIAN_POINT ( 'NONE',  ( 105.0000000000000000, 0.000000000000000000, 59.99999999999999289 ) ) ;
#24302=CARTESIAN_POINT ( 'NONE',  ( -19.65312891409030271, 5.000000000000004441, 54.99999999999999289 ) ) ;
#24383=DIRECTION ( 'NONE',  ( -1.000000000000000000, 0.000000000000000000, 0.000000000000000000 ) ) ;
#24433=LINE ( 'NONE', #8731, #22382 ) ;
#24442=DIRECTION ( 'NONE',  ( -1.000000000000000000, 0.000000000000000000, 0.000000000000000000 ) ) ;
#24472=ADVANCED_FACE ( 'NONE', ( #16419 ), #32112, .T. ) ;
#24485=LINE ( 'NONE', #71611, #58200 ) ;
#24525=EDGE_LOOP ( 'NONE', ( #67490, #27853, #71668, #70362, #19219, #27737, #75345, #85335 ) ) ;
#24538=EDGE_CURVE ( 'NONE', #65750, #14428, #33640, .T. ) ;
#24562=CYLINDRICAL_SURFACE ( 'NONE', #86341, 14.21260523776213347 ) ;
#24643=ORIENTED_EDGE ( 'NONE', *, *, #61740, .F. ) ;
#24689=CARTESIAN_POINT ( 'NONE',  ( -110.0000000000000142, -8.000000000000000000, 9.212605237762145904 ) ) ;
#24712=FACE_OUTER_BOUND ( 'NONE', #57399, .T. ) ;
#24734=EDGE_CURVE ( 'NONE', #29494, #87383, #3743, .T. ) ;
#24735=CIRCLE ( 'NONE', #53782, 7.499999999999996447 ) ;
#24746=ORIENTED_EDGE ( 'NONE', *, *, #10004, .F. ) ;
#24789=ORIENTED_EDGE ( 'NONE', *, *, #75799, .T. ) ;
#24793=DIRECTION ( 'NONE',  ( 1.000000000000000000, 0.000000000000000000, 0.000000000000000000 ) ) ;
#24857=FACE_OUTER_BOUND ( 'NONE', #97107, .T. ) ;
#24906=VERTEX_POINT ( 'NONE', #14802 ) ;
#24949=CARTESIAN_POINT ( 'NONE',  ( -13.11024591527734628, 6.000000000000000000, 32.50000000000000000 ) ) ;
#24976=EDGE_CURVE ( 'NONE', #24906, #37352, #63901, .T. ) ;
#25144=DIRECTION ( 'NONE',  ( -0.000000000000000000, -0.000000000000000000, -1.000000000000000000 ) ) ;
#25174=AXIS2_PLACEMENT_3D ( 'NONE', #63247, #82500, #43924 ) ;
#25237=ORIENTED_EDGE ( 'NONE', *, *, #58367, .T. ) ;
#25362=CARTESIAN_POINT ( 'NONE',  ( 110.0000000000000000, -8.000000000000000000, 9.212605237762131694 ) ) ;
#25438=AXIS2_PLACEMENT_3D ( 'NONE', #35755, #4874, #28153 ) ;
#25457=DIRECTION ( 'NONE',  ( 1.000000000000000000, 0.000000000000000000, 0.000000000000000000 ) ) ;
#25645=ORIENTED_EDGE ( 'NONE', *, *, #88683, .T. ) ;
#25707=DIRECTION ( 'NONE',  ( 0.000000000000000000, 1.000000000000000000, 0.000000000000000000 ) ) ;
#25754=ORIENTED_EDGE ( 'NONE', *, *, #50687, .T. ) ;
#25855=DIRECTION ( 'NONE',  ( -0.000000000000000000, -0.000000000000000000, 1.000000000000000000 ) ) ;
#25867=VECTOR ( 'NONE', #49329, 1000.000000000000000 ) ;
#25881=DIRECTION ( 'NONE',  ( 0.000000000000000000, 0.000000000000000000, -1.000000000000000000 ) ) ;
#25887=DIRECTION ( 'NONE',  ( 1.082076799516502080E-16, 0.000000000000000000, 1.000000000000000000 ) ) ;
#25923=DIRECTION ( 'NONE',  ( 0.000000000000000000, 0.000000000000000000, 1.000000000000000000 ) ) ;
#25927=( NAMED_UNIT ( * ) PLANE_ANGLE_UNIT ( ) SI_UNIT ( $, .RADIAN. ) );
#26033=ORIENTED_EDGE ( 'NONE', *, *, #49173, .T. ) ;
#26078=CARTESIAN_POINT ( 'NONE',  ( -13.11024591527723615, 27.99999999999999645, -40.00000000000016342 ) ) ;
#26101=DIRECTION ( 'NONE',  ( 1.000000000000000000, 1.804112415015878984E-15, 0.000000000000000000 ) ) ;
#26170=CARTESIAN_POINT ( 'NONE',  ( -110.0000000000000000, 0.000000000000000000, 9.212605237762156563 ) ) ;
#26184=EDGE_CURVE ( 'NONE', #3825, #63991, #85045, .T. ) ;
#26226=DIRECTION ( 'NONE',  ( -1.000000000000000000, -1.156482317317871133E-15, 0.000000000000000000 ) ) ;
#26267=DIRECTION ( 'NONE',  ( 0.000000000000000000, 1.000000000000000000, 0.000000000000000000 ) ) ;
#26271=DIRECTION ( 'NONE',  ( 1.000000000000000000, 0.000000000000000000, 0.000000000000000000 ) ) ;
#26308=DIRECTION ( 'NONE',  ( 0.000000000000000000, 1.000000000000000000, 0.000000000000000000 ) ) ;
#26347=VECTOR ( 'NONE', #63981, 1000.000000000000000 ) ;
#26392=ORIENTED_EDGE ( 'NONE', *, *, #7187, .F. ) ;
#26434=CIRCLE ( 'NONE', #7024, 9.212605237762131694 ) ;
#26493=LINE ( 'NONE', #57370, #3315 ) ;
#26524=ORIENTED_EDGE ( 'NONE', *, *, #81797, .T. ) ;
#26545=VERTEX_POINT ( 'NONE', #53572 ) ;
#26592=EDGE_LOOP ( 'NONE', ( #84019, #83843, #27679, #86744, #54931, #43798, #33492, #83443 ) ) ;
#26644=CARTESIAN_POINT ( 'NONE',  ( 51.80235952159637236, 80.00000000000000000, -10.00000000000000178 ) ) ;
#26649=AXIS2_PLACEMENT_3D ( 'NONE', #66506, #32437, #88695 ) ;
#26729=DIRECTION ( 'NONE',  ( -0.000000000000000000, -1.000000000000000000, -0.000000000000000000 ) ) ;
#26759=LINE ( 'NONE', #57642, #79750 ) ;
#26764=EDGE_CURVE ( 'NONE', #8604, #65750, #36630, .T. ) ;
#26781=AXIS2_PLACEMENT_3D ( 'NONE', #77934, #55595, #86578 ) ;
#26782=ORIENTED_EDGE ( 'NONE', *, *, #24538, .F. ) ;
#26844=ADVANCED_FACE ( 'NONE', ( #74677 ), #89889, .F. ) ;
#26923=CARTESIAN_POINT ( 'NONE',  ( 105.0000000000000000, 4.999999999999999112, -54.99999999999999289 ) ) ;
#26964=CARTESIAN_POINT ( 'NONE',  ( -110.0000000000000000, 0.000000000000000000, 59.99999999999999289 ) ) ;
#26978=DIRECTION ( 'NONE',  ( 0.000000000000000000, -1.000000000000000000, 0.000000000000000000 ) ) ;
#26985=VECTOR ( 'NONE', #33044, 1000.000000000000000 ) ;
#27008=ADVANCED_FACE ( 'NONE', ( #30369 ), #61252, .T. ) ;
#27034=DIRECTION ( 'NONE',  ( 0.8660254037844378194, 0.5000000000000015543, -0.000000000000000000 ) ) ;
#27050=ORIENTED_EDGE ( 'NONE', *, *, #91613, .T. ) ;
#27092=ORIENTED_EDGE ( 'NONE', *, *, #47470, .T. ) ;
#27131=ORIENTED_EDGE ( 'NONE', *, *, #89441, .T. ) ;
#27144=CARTESIAN_POINT ( 'NONE',  ( 84.99999999999997158, 27.49999999999999645, 59.99999999999999289 ) ) ;
#27204=DIRECTION ( 'NONE',  ( 1.000000000000000000, 0.000000000000000000, 0.000000000000000000 ) ) ;
#27210=EDGE_CURVE ( 'NONE', #79692, #48169, #20685, .T. ) ;
#27243=VERTEX_POINT ( 'NONE', #75898 ) ;
#27257=ORIENTED_EDGE ( 'NONE', *, *, #81547, .F. ) ;
#27260=VECTOR ( 'NONE', #85446, 1000.000000000000000 ) ;
#27347=CARTESIAN_POINT ( 'NONE',  ( -51.42721978966704910, 42.16899896210639298, 10.00000000000001599 ) ) ;
#27382=VECTOR ( 'NONE', #49004, 1000.000000000000000 ) ;
#27388=EDGE_LOOP ( 'NONE', ( #95326, #90624, #74306, #59517 ) ) ;
#27407=LINE ( 'NONE', #97321, #22174 ) ;
#27429=DIRECTION ( 'NONE',  ( 0.000000000000000000, -0.000000000000000000, 1.000000000000000000 ) ) ;
#27455=AXIS2_PLACEMENT_3D ( 'NONE', #6812, #89957, #6316 ) ;
#27524=EDGE_CURVE ( 'NONE', #69092, #61410, #38348, .T. ) ;
#27545=EDGE_LOOP ( 'NONE', ( #55657, #40291, #69856, #44904, #13538, #52069, #46453, #68741, #67627, #31572, #57149 ) ) ;
#27556=AXIS2_PLACEMENT_3D ( 'NONE', #78639, #34039, #71540 ) ;
#27575=CARTESIAN_POINT ( 'NONE',  ( 110.0000000000000000, 0.000000000000000000, 59.99999999999999289 ) ) ;
#27633=ORIENTED_EDGE ( 'NONE', *, *, #306, .F. ) ;
#27636=CARTESIAN_POINT ( 'NONE',  ( -110.0000000000000142, -8.000000000000000000, -14.21260523776211926 ) ) ;
#27679=ORIENTED_EDGE ( 'NONE', *, *, #68895, .F. ) ;
#27733=CARTESIAN_POINT ( 'NONE',  ( -13.11024591527734628, 6.000000000000000000, 32.50000000000000000 ) ) ;
#27737=ORIENTED_EDGE ( 'NONE', *, *, #1001, .F. ) ;
#27770=ORIENTED_EDGE ( 'NONE', *, *, #15724, .T. ) ;
#27816=CARTESIAN_POINT ( 'NONE',  ( 48.91560817564824504, 80.00000000000000000, 54.99999999999999289 ) ) ;
#27852=AXIS2_PLACEMENT_3D ( 'NONE', #27733, #26729, #18136 ) ;
#27853=ORIENTED_EDGE ( 'NONE', *, *, #35519, .F. ) ;
#27923=DIRECTION ( 'NONE',  ( 0.000000000000000000, -1.000000000000000000, 0.000000000000000000 ) ) ;
#27924=LINE ( 'NONE', #58807, #61254 ) ;
#27967=DIRECTION ( 'NONE',  ( -0.000000000000000000, -1.000000000000000000, -0.000000000000000000 ) ) ;
#27988=AXIS2_PLACEMENT_3D ( 'NONE', #91920, #45753, #94279 ) ;
#28007=CARTESIAN_POINT ( 'NONE',  ( 61.15274061880273848, 58.80466486950705729, 0.000000000000000000 ) ) ;
#28013=AXIS2_PLACEMENT_3D ( 'NONE', #95170, #58113, #89094 ) ;
#28070=LINE ( 'NONE', #74705, #59131 ) ;
#28077=EDGE_CURVE ( 'NONE', #57607, #75521, #71912, .T. ) ;
#28153=DIRECTION ( 'NONE',  ( 0.000000000000000000, 0.000000000000000000, 1.000000000000000000 ) ) ;
#28168=PRODUCT_DEFINITION_SHAPE ( 'NONE', 'NONE',  #71293 ) ;
#28228=CARTESIAN_POINT ( 'NONE',  ( 49.65150239490934325, 78.72539382324355017, 10.00000000000000178 ) ) ;
#28280=CARTESIAN_POINT ( 'NONE',  ( -19.65312891409030271, 93.06504152958497400, -10.00000000000000000 ) ) ;
#28291=VECTOR ( 'NONE', #51773, 1000.000000000000114 ) ;
#28336=CARTESIAN_POINT ( 'NONE',  ( 79.99999999999998579, 9.999999999999985789, 59.99999999999999289 ) ) ;
#28355=PLANE ( 'NONE',  #29737 ) ;
#28379=CARTESIAN_POINT ( 'NONE',  ( 105.0000000000000000, 10.00000000000003197, 59.99999999999999289 ) ) ;
#28394=EDGE_LOOP ( 'NONE', ( #84395, #69704, #27770, #88347 ) ) ;
#28396=ORIENTED_EDGE ( 'NONE', *, *, #19107, .F. ) ;
#28399=CIRCLE ( 'NONE', #41343, 60.00000000000001421 ) ;
#28403=VERTEX_POINT ( 'NONE', #58019 ) ;
#28416=CARTESIAN_POINT ( 'NONE',  ( -13.11024591527734628, 0.000000000000000000, 32.50000000000000000 ) ) ;
#28462=EDGE_LOOP ( 'NONE', ( #53706, #12666, #47797, #4851, #87726, #37210, #59606, #10581 ) ) ;
#28511=ORIENTED_EDGE ( 'NONE', *, *, #18971, .F. ) ;
#28531=CARTESIAN_POINT ( 'NONE',  ( 39.80235952159635815, 84.99999999999998579, 59.99999999999999289 ) ) ;
#28539=CARTESIAN_POINT ( 'NONE',  ( 79.99999999999997158, 26.16025403784438907, 54.99999999999999289 ) ) ;
#28589=DIRECTION ( 'NONE',  ( 0.8660254037844379305, 0.5000000000000015543, 0.000000000000000000 ) ) ;
#28594=ORIENTED_EDGE ( 'NONE', *, *, #1001, .T. ) ;
#28606=VECTOR ( 'NONE', #28881, 1000.000000000000000 ) ;
#28624=PLANE ( 'NONE',  #83140 ) ;
#28651=ADVANCED_FACE ( 'NONE', ( #77600 ), #8186, .F. ) ;
#28789=EDGE_CURVE ( 'NONE', #75521, #58073, #58271, .T. ) ;
#28847=FACE_OUTER_BOUND ( 'NONE', #9432, .T. ) ;
#28863=LINE ( 'NONE', #51664, #90286 ) ;
#28868=AXIS2_PLACEMENT_3D ( 'NONE', #97172, #20639, #89583 ) ;
#28881=DIRECTION ( 'NONE',  ( -0.000000000000000000, -1.000000000000000000, -0.000000000000000000 ) ) ;
#28882=VECTOR ( 'NONE', #14229, 1000.000000000000000 ) ;
#28924=AXIS2_PLACEMENT_3D ( 'NONE', #13798, #21408, #29016 ) ;
#28939=EDGE_CURVE ( 'NONE', #31618, #2827, #6070, .T. ) ;
#28967=CIRCLE ( 'NONE', #96913, 60.00000000000002132 ) ;
#28973=AXIS2_PLACEMENT_3D ( 'NONE', #28280, #36883, #52082 ) ;
#28991=AXIS2_PLACEMENT_3D ( 'NONE', #86861, #94433, #23989 ) ;
#29016=DIRECTION ( 'NONE',  ( 0.000000000000000000, 0.000000000000000000, -1.000000000000000000 ) ) ;
#29018=ORIENTED_EDGE ( 'NONE', *, *, #15629, .T. ) ;
#29119=CARTESIAN_POINT ( 'NONE',  ( -13.11024591527734628, 27.99999999999999645, 32.50000000000000000 ) ) ;
#29165=EDGE_CURVE ( 'NONE', #80375, #43945, #64266, .T. ) ;
#29184=LINE ( 'NONE', #91015, #75663 ) ;
#29213=LINE ( 'NONE', #60081, #42873 ) ;
#29425=LINE ( 'NONE', #37507, #28882 ) ;
#29464=ORIENTED_EDGE ( 'NONE', *, *, #97587, .F. ) ;
#29469=EDGE_CURVE ( 'NONE', #44408, #97401, #80441, .T. ) ;
#29475=ADVANCED_FACE ( 'NONE', ( #74136, #81754 ), #82266, .T. ) ;
#29494=VERTEX_POINT ( 'NONE', #28007 ) ;
#29737=AXIS2_PLACEMENT_3D ( 'NONE', #59232, #20781, #15638 ) ;
#29773=EDGE_CURVE ( 'NONE', #97093, #87466, #27407, .T. ) ;
#29785=PLANE ( 'NONE',  #46746 ) ;
#29800=CARTESIAN_POINT ( 'NONE',  ( 105.0000000000000000, 10.00000000000003197, 59.99999999999999289 ) ) ;
#29812=DIRECTION ( 'NONE',  ( -1.000000000000000000, 0.000000000000000000, 0.000000000000000000 ) ) ;
#29896=ADVANCED_FACE ( 'NONE', ( #71309, #39366 ), #94130, .F. ) ;
#29910=DIRECTION ( 'NONE',  ( 0.000000000000000000, 0.000000000000000000, 1.000000000000000000 ) ) ;
#30142=DIRECTION ( 'NONE',  ( 0.000000000000000000, 0.000000000000000000, -1.000000000000000000 ) ) ;
#30230=VECTOR ( 'NONE', #54668, 1000.000000000000000 ) ;
#30233=ORIENTED_EDGE ( 'NONE', *, *, #69475, .T. ) ;
#30260=ORIENTED_EDGE ( 'NONE', *, *, #43573, .T. ) ;
#30276=CARTESIAN_POINT ( 'NONE',  ( -13.11024591527723615, 27.99999999999999645, -32.50000000000017053 ) ) ;
#30330=VERTEX_POINT ( 'NONE', #26078 ) ;
#30369=FACE_OUTER_BOUND ( 'NONE', #13666, .T. ) ;
#30395=DIRECTION ( 'NONE',  ( 1.000000000000000000, 0.000000000000000000, -1.082076799516502204E-16 ) ) ;
#30569=VECTOR ( 'NONE', #63115, 1000.000000000000000 ) ;
#30588=DIRECTION ( 'NONE',  ( -1.000000000000000000, -1.156482317317871133E-15, 0.000000000000000000 ) ) ;
#30635=CARTESIAN_POINT ( 'NONE',  ( 79.99999999999998579, 9.999999999999985789, -54.99999999999999289 ) ) ;
#30686=LINE ( 'NONE', #23062, #50704 ) ;
#30735=DIRECTION ( 'NONE',  ( -0.000000000000000000, 1.000000000000000000, 0.000000000000000000 ) ) ;
#30784=DIRECTION ( 'NONE',  ( 0.000000000000000000, -0.000000000000000000, 1.000000000000000000 ) ) ;
#30852=EDGE_CURVE ( 'NONE', #48169, #55924, #98110, .T. ) ;
#30906=ORIENTED_EDGE ( 'NONE', *, *, #21787, .F. ) ;
#30907=CARTESIAN_POINT ( 'NONE',  ( -110.0000000000000142, -8.000000000000000000, -9.212605237762117483 ) ) ;
#30931=DIRECTION ( 'NONE',  ( -0.000000000000000000, -1.000000000000000000, -0.000000000000000000 ) ) ;
#30964=EDGE_LOOP ( 'NONE', ( #53773, #60367, #38575, #24233, #75980, #60507, #33091, #37118, #75665, #95309, #84891, #58327 ) ) ;
#31032=PLANE ( 'NONE',  #80691 ) ;
#31067=ORIENTED_EDGE ( 'NONE', *, *, #73888, .F. ) ;
#31110=ORIENTED_EDGE ( 'NONE', *, *, #1638, .T. ) ;
#31115=DIRECTION ( 'NONE',  ( -0.5000000000000011102, -0.8660254037844380415, 0.000000000000000000 ) ) ;
#31138=CARTESIAN_POINT ( 'NONE',  ( 49.80235952159635815, 85.00000000000000000, -10.00000000000000000 ) ) ;
#31177=CARTESIAN_POINT ( 'NONE',  ( 18.52134341065868384, 22.64441083166259716, 0.000000000000000000 ) ) ;
#31343=ORIENTED_EDGE ( 'NONE', *, *, #2190, .T. ) ;
#31393=LINE ( 'NONE', #76517, #64469 ) ;
#31406=EDGE_CURVE ( 'NONE', #57607, #42192, #39349, .T. ) ;
#31417=CARTESIAN_POINT ( 'NONE',  ( -65.66987298107781612, 17.49999999999999645, 59.99999999999999289 ) ) ;
#31434=LINE ( 'NONE', #62328, #68546 ) ;
#31497=EDGE_LOOP ( 'NONE', ( #60724, #5969, #99816, #46740 ) ) ;
#31505=ORIENTED_EDGE ( 'NONE', *, *, #10886, .T. ) ;
#31510=CARTESIAN_POINT ( 'NONE',  ( 110.0000000000000000, 0.000000000000000000, -9.212605237762131694 ) ) ;
#31536=LINE ( 'NONE', #46744, #26985 ) ;
#31572=ORIENTED_EDGE ( 'NONE', *, *, #40587, .F. ) ;
#31593=VECTOR ( 'NONE', #61374, 1000.000000000000000 ) ;
#31600=EDGE_CURVE ( 'NONE', #51782, #100286, #6739, .T. ) ;
#31618=VERTEX_POINT ( 'NONE', #84278 ) ;
#31646=APPLICATION_CONTEXT ( 'automotive_design' ) ;
#31649=LINE ( 'NONE', #15966, #50846 ) ;
#31771=AXIS2_PLACEMENT_3D ( 'NONE', #39054, #17276, #24383 ) ;
#31830=EDGE_LOOP ( 'NONE', ( #9368, #49025, #53281, #62337 ) ) ;
#31853=AXIS2_PLACEMENT_3D ( 'NONE', #98901, #79118, #2594 ) ;
#31854=VERTEX_POINT ( 'NONE', #50710 ) ;
#31863=EDGE_CURVE ( 'NONE', #33601, #3825, #95881, .T. ) ;
#31866=VECTOR ( 'NONE', #30395, 1000.000000000000000 ) ;
#31869=VERTEX_POINT ( 'NONE', #66911 ) ;
#31876=AXIS2_PLACEMENT_3D ( 'NONE', #57140, #88121, #61123 ) ;
#31996=VECTOR ( 'NONE', #42297, 1000.000000000000000 ) ;
#32007=ADVANCED_FACE ( 'NONE', ( #75528, #6622 ), #68898, .F. ) ;
#32013=VECTOR ( 'NONE', #69348, 1000.000000000000000 ) ;
#32045=EDGE_CURVE ( 'NONE', #87128, #91430, #4463, .T. ) ;
#32057=CYLINDRICAL_SURFACE ( 'NONE', #56512, 9.212605237762131694 ) ;
#32067=VECTOR ( 'NONE', #57777, 1000.000000000000000 ) ;
#32076=AXIS2_PLACEMENT_3D ( 'NONE', #70486, #1615, #55761 ) ;
#32100=ADVANCED_FACE ( 'NONE', ( #38993 ), #16208, .F. ) ;
#32112=PLANE ( 'NONE',  #91717 ) ;
#32139=VECTOR ( 'NONE', #4873, 1000.000000000000000 ) ;
#32181=LINE ( 'NONE', #94029, #3924 ) ;
#32220=CARTESIAN_POINT ( 'NONE',  ( -13.11024591527723615, 15.00000000000000000, -32.50000000000017053 ) ) ;
#32249=LINE ( 'NONE', #79897, #10765 ) ;
#32252=CARTESIAN_POINT ( 'NONE',  ( -19.65312891409030271, 93.06504152958497400, 10.00000000000000000 ) ) ;
#32256=ORIENTED_EDGE ( 'NONE', *, *, #97587, .T. ) ;
#32326=ORIENTED_EDGE ( 'NONE', *, *, #8589, .T. ) ;
#32393=CARTESIAN_POINT ( 'NONE',  ( -105.0000000000000000, 4.999999999999999112, -54.99999999999999289 ) ) ;
#32437=DIRECTION ( 'NONE',  ( -0.000000000000000000, -1.000000000000000000, -0.000000000000000000 ) ) ;
#32489=VERTEX_POINT ( 'NONE', #93074 ) ;
#32503=EDGE_LOOP ( 'NONE', ( #67993, #74902, #31505, #45077 ) ) ;
#32600=LINE ( 'NONE', #39170, #89612 ) ;
#32657=CARTESIAN_POINT ( 'NONE',  ( 71.15274061880276690, 41.48415679381830046, 1.224646799147354045E-15 ) ) ;
#32679=ADVANCED_FACE ( 'NONE', ( #63528 ), #63029, .T. ) ;
#32767=VERTEX_POINT ( 'NONE', #49340 ) ;
#32835=AXIS2_PLACEMENT_3D ( 'NONE', #88441, #19001, #49876 ) ;
#32857=DIRECTION ( 'NONE',  ( -0.000000000000000000, -0.000000000000000000, -1.000000000000000000 ) ) ;
#32945=CYLINDRICAL_SURFACE ( 'NONE', #21314, 60.00000000000002132 ) ;
#33044=DIRECTION ( 'NONE',  ( -0.000000000000000000, -0.000000000000000000, -1.000000000000000000 ) ) ;
#33091=ORIENTED_EDGE ( 'NONE', *, *, #14525, .T. ) ;
#33154=UNCERTAINTY_MEASURE_WITH_UNIT (LENGTH_MEASURE( 1.000000000000000082E-05 ), #20316, 'distance_accuracy_value', 'NONE');
#33191=DIRECTION ( 'NONE',  ( 1.804112415015878984E-15, -1.000000000000000000, 0.000000000000000000 ) ) ;
#33230=LINE ( 'NONE', #79880, #60530 ) ;
#33232=ORIENTED_EDGE ( 'NONE', *, *, #30852, .T. ) ;
#33261=VERTEX_POINT ( 'NONE', #28531 ) ;
#33294=ADVANCED_FACE ( 'NONE', ( #41740 ), #3763, .T. ) ;
#33313=CARTESIAN_POINT ( 'NONE',  ( 110.0000000000000000, 15.00000000000000000, 9.212605237762131694 ) ) ;
#33343=VERTEX_POINT ( 'NONE', #66544 ) ;
#33364=EDGE_LOOP ( 'NONE', ( #18666, #84868, #14468, #54363 ) ) ;
#33465=CARTESIAN_POINT ( 'NONE',  ( -13.11024591527723615, 27.99999999999999645, -48.00000000000017053 ) ) ;
#33466=LINE ( 'NONE', #95817, #80894 ) ;
#33467=CARTESIAN_POINT ( 'NONE',  ( -13.11024591527734628, 15.00000000000000000, 32.50000000000000000 ) ) ;
#33482=FACE_OUTER_BOUND ( 'NONE', #70421, .T. ) ;
#33492=ORIENTED_EDGE ( 'NONE', *, *, #11761, .T. ) ;
#33500=DIRECTION ( 'NONE',  ( 0.000000000000000000, 0.000000000000000000, -1.000000000000000000 ) ) ;
#33501=AXIS2_PLACEMENT_3D ( 'NONE', #19048, #73236, #33740 ) ;
#33555=EDGE_CURVE ( 'NONE', #79692, #37942, #24433, .T. ) ;
#33574=DIRECTION ( 'NONE',  ( 0.000000000000000000, 0.000000000000000000, -1.000000000000000000 ) ) ;
#33601=VERTEX_POINT ( 'NONE', #23415 ) ;
#33625=CARTESIAN_POINT ( 'NONE',  ( -19.65312891409030271, 93.06504152958497400, 10.00000000000000000 ) ) ;
#33640=LINE ( 'NONE', #94967, #17260 ) ;
#33740=DIRECTION ( 'NONE',  ( 0.000000000000000000, 0.000000000000000000, 1.000000000000000000 ) ) ;
#33839=ORIENTED_EDGE ( 'NONE', *, *, #77682, .F. ) ;
#33848=EDGE_LOOP ( 'NONE', ( #64503, #62916, #50179, #50626, #90066 ) ) ;
#33876=ORIENTED_EDGE ( 'NONE', *, *, #68895, .T. ) ;
#33902=DIRECTION ( 'NONE',  ( 1.110223024625156343E-15, -1.000000000000000000, 0.000000000000000000 ) ) ;
#33913=ORIENTED_EDGE ( 'NONE', *, *, #64126, .T. ) ;
#33923=VECTOR ( 'NONE', #20172, 1000.000000000000000 ) ;
#34039=DIRECTION ( 'NONE',  ( -0.000000000000000000, -0.000000000000000000, -1.000000000000000000 ) ) ;
#34203=DIRECTION ( 'NONE',  ( 0.000000000000000000, 1.000000000000000000, 0.000000000000000000 ) ) ;
#34225=FACE_OUTER_BOUND ( 'NONE', #10345, .T. ) ;
#34260=CIRCLE ( 'NONE', #60117, 10.00000000000001066 ) ;
#34316=VERTEX_POINT ( 'NONE', #19321 ) ;
#34351=ORIENTED_EDGE ( 'NONE', *, *, #80926, .T. ) ;
#34361=CARTESIAN_POINT ( 'NONE',  ( -70.00000000000000000, 20.00000000000000000, 59.99999999999999289 ) ) ;
#34367=ORIENTED_EDGE ( 'NONE', *, *, #45399, .T. ) ;
#34434=EDGE_CURVE ( 'NONE', #51782, #36590, #56368, .T. ) ;
#34486=CARTESIAN_POINT ( 'NONE',  ( 105.0000000000000000, 0.000000000000000000, 14.21260523776213347 ) ) ;
#34534=CARTESIAN_POINT ( 'NONE',  ( 48.91560817564824504, 80.00000000000000000, -10.00000000000000178 ) ) ;
#34536=ADVANCED_FACE ( 'NONE', ( #65259 ), #79510, .F. ) ;
#34580=CARTESIAN_POINT ( 'NONE',  ( -110.0000000000000142, 15.00000000000000000, -9.212605237762117483 ) ) ;
#34645=DIRECTION ( 'NONE',  ( 0.000000000000000000, 0.000000000000000000, -1.000000000000000000 ) ) ;
#34691=ORIENTED_EDGE ( 'NONE', *, *, #78170, .F. ) ;
#34988=CARTESIAN_POINT ( 'NONE',  ( 93.96857342517719758, 15.00000000000000000, 0.000000000000000000 ) ) ;
#34995=CARTESIAN_POINT ( 'NONE',  ( 109.9999999999999716, 10.00000000000004086, 14.21260523776213347 ) ) ;
#34998=ORIENTED_EDGE ( 'NONE', *, *, #78809, .F. ) ;
#35004=CARTESIAN_POINT ( 'NONE',  ( -110.0000000000000000, 0.000000000000000000, 59.99999999999999289 ) ) ;
#35032=VECTOR ( 'NONE', #10076, 1000.000000000000000 ) ;
#35069=DIRECTION ( 'NONE',  ( 0.000000000000000000, 1.000000000000000000, 0.000000000000000000 ) ) ;
#35095=LINE ( 'NONE', #95958, #97945 ) ;
#35154=VECTOR ( 'NONE', #91513, 1000.000000000000000 ) ;
#35186=CARTESIAN_POINT ( 'NONE',  ( 105.0000000000000142, 93.06504152958497400, 54.99999999999999289 ) ) ;
#35258=CIRCLE ( 'NONE', #40076, 12.50000000000000000 ) ;
#35306=VERTEX_POINT ( 'NONE', #47080 ) ;
#35308=CARTESIAN_POINT ( 'NONE',  ( -110.0000000000000142, 10.00000000000000178, -14.21260523776211926 ) ) ;
#35325=EDGE_CURVE ( 'NONE', #6085, #13462, #23269, .T. ) ;
#35374=ADVANCED_FACE ( 'NONE', ( #95620 ), #41851, .T. ) ;
#35437=ORIENTED_EDGE ( 'NONE', *, *, #59092, .F. ) ;
#35445=LINE ( 'NONE', #28336, #86430 ) ;
#35487=VECTOR ( 'NONE', #82359, 1000.000000000000000 ) ;
#35512=ORIENTED_EDGE ( 'NONE', *, *, #46263, .T. ) ;
#35519=EDGE_CURVE ( 'NONE', #87466, #1591, #89041, .T. ) ;
#35529=CARTESIAN_POINT ( 'NONE',  ( 110.0000000000000000, 0.000000000000000000, 59.99999999999999289 ) ) ;
#35540=VECTOR ( 'NONE', #77014, 999.9999999999998863 ) ;
#35593=ORIENTED_EDGE ( 'NONE', *, *, #46065, .T. ) ;
#35608=FACE_OUTER_BOUND ( 'NONE', #70609, .T. ) ;
#35612=DIRECTION ( 'NONE',  ( 0.000000000000000000, 0.000000000000000000, 1.000000000000000000 ) ) ;
#35648=CARTESIAN_POINT ( 'NONE',  ( -70.00000000000000000, 20.00000000000000000, 59.99999999999999289 ) ) ;
#35652=EDGE_CURVE ( 'NONE', #16631, #20674, #7210, .T. ) ;
#35684=CARTESIAN_POINT ( 'NONE',  ( 51.80235952159636525, 85.00000000000000000, -59.99999999999999289 ) ) ;
#35736=CARTESIAN_POINT ( 'NONE',  ( 84.99999999999997158, 27.49999999999999645, -59.99999999999999289 ) ) ;
#35755=CARTESIAN_POINT ( 'NONE',  ( -13.11024591527734628, 4.999999999999999112, 32.50000000000000000 ) ) ;
#35859=VERTEX_POINT ( 'NONE', #26923 ) ;
#35883=ADVANCED_FACE ( 'NONE', ( #88781, #19351, #42594 ), #96861, .F. ) ;
#35914=DIRECTION ( 'NONE',  ( 0.000000000000000000, 0.000000000000000000, -1.000000000000000000 ) ) ;
#35942=VECTOR ( 'NONE', #27967, 1000.000000000000000 ) ;
#35948=ORIENTED_EDGE ( 'NONE', *, *, #8799, .T. ) ;
#35972=SHAPE_REPRESENTATION ( 'Lower Tilting Cradle Base Segment', ( #68784 ), #2502 ) ;
#36181=CARTESIAN_POINT ( 'NONE',  ( -86.81108781737714253, 10.00000000000000178, 0.000000000000000000 ) ) ;
#36191=ORIENTED_EDGE ( 'NONE', *, *, #35652, .T. ) ;
#36200=DIRECTION ( 'NONE',  ( -5.984665299743594308E-16, 0.000000000000000000, -1.000000000000000000 ) ) ;
#36246=VERTEX_POINT ( 'NONE', #73410 ) ;
#36257=ORIENTED_EDGE ( 'NONE', *, *, #38257, .F. ) ;
#36288=EDGE_CURVE ( 'NONE', #24906, #100286, #75404, .T. ) ;
#36331=ADVANCED_FACE ( 'NONE', ( #84523 ), #74909, .T. ) ;
#36332=CARTESIAN_POINT ( 'NONE',  ( 110.0000000000000000, -8.000000000000000000, 14.21260523776213347 ) ) ;
#36333=ADVANCED_FACE ( 'NONE', ( #82546 ), #29785, .T. ) ;
#36435=ORIENTED_EDGE ( 'NONE', *, *, #26184, .T. ) ;
#36474=CARTESIAN_POINT ( 'NONE',  ( -13.11024591527734628, 6.000000000000000000, 20.00000000000000000 ) ) ;
#36590=VERTEX_POINT ( 'NONE', #41877 ) ;
#36630=LINE ( 'NONE', #35648, #67292 ) ;
#36631=CARTESIAN_POINT ( 'NONE',  ( -13.11024591527734628, 0.000000000000000000, 20.00000000000000000 ) ) ;
#36680=PLANE ( 'NONE',  #86095 ) ;
#36717=AXIS2_PLACEMENT_3D ( 'NONE', #49452, #40337, #87538 ) ;
#36740=VECTOR ( 'NONE', #26978, 1000.000000000000000 ) ;
#36788=LINE ( 'NONE', #22091, #51622 ) ;
#36834=LINE ( 'NONE', #82504, #43205 ) ;
#36865=ORIENTED_EDGE ( 'NONE', *, *, #88365, .T. ) ;
#36883=DIRECTION ( 'NONE',  ( 0.000000000000000000, 0.000000000000000000, 1.000000000000000000 ) ) ;
#36947=LINE ( 'NONE', #453, #32013 ) ;
#36953=DIRECTION ( 'NONE',  ( 0.000000000000000000, 1.000000000000000000, 0.000000000000000000 ) ) ;
#37054=VECTOR ( 'NONE', #76405, 1000.000000000000000 ) ;
#37118=ORIENTED_EDGE ( 'NONE', *, *, #91055, .T. ) ;
#37138=LINE ( 'NONE', #91378, #48243 ) ;
#37199=VECTOR ( 'NONE', #47193, 1000.000000000000227 ) ;
#37210=ORIENTED_EDGE ( 'NONE', *, *, #82047, .T. ) ;
#37313=EDGE_LOOP ( 'NONE', ( #35437, #25645, #85730, #64308 ) ) ;
#37328=CARTESIAN_POINT ( 'NONE',  ( -13.11024591527734451, 27.99999999999999645, 40.00000000000000000 ) ) ;
#37352=VERTEX_POINT ( 'NONE', #57979 ) ;
#37357=ORIENTED_EDGE ( 'NONE', *, *, #19107, .T. ) ;
#37375=EDGE_CURVE ( 'NONE', #5700, #26545, #17463, .T. ) ;
#37410=VECTOR ( 'NONE', #100116, 1000.000000000000000 ) ;
#37494=EDGE_CURVE ( 'NONE', #54703, #31618, #35258, .T. ) ;
#37496=DIRECTION ( 'NONE',  ( -0.000000000000000000, 1.000000000000000000, 0.000000000000000000 ) ) ;
#37507=CARTESIAN_POINT ( 'NONE',  ( 38.90713653809340400, 79.99999999999998579, 54.99999999999999289 ) ) ;
#37558=ORIENTED_EDGE ( 'NONE', *, *, #88112, .F. ) ;
#37610=EDGE_CURVE ( 'NONE', #27243, #57163, #64973, .T. ) ;
#37647=EDGE_LOOP ( 'NONE', ( #16986, #48454 ) ) ;
#37785=LINE ( 'NONE', #99619, #27260 ) ;
#37922=CARTESIAN_POINT ( 'NONE',  ( 48.91560817564824504, 80.00000000000000000, 59.99999999999999289 ) ) ;
#37928=ORIENTED_EDGE ( 'NONE', *, *, #60227, .T. ) ;
#37942=VERTEX_POINT ( 'NONE', #27347 ) ;
#38039=CYLINDRICAL_SURFACE ( 'NONE', #54930, 12.49999999999999645 ) ;
#38041=ORIENTED_EDGE ( 'NONE', *, *, #91233, .F. ) ;
#38156=VERTEX_POINT ( 'NONE', #79433 ) ;
#38194=ORIENTED_EDGE ( 'NONE', *, *, #46570, .F. ) ;
#38257=EDGE_CURVE ( 'NONE', #47538, #87383, #54679, .T. ) ;
#38348=LINE ( 'NONE', #92601, #68944 ) ;
#38370=DIRECTION ( 'NONE',  ( 0.8575671445351807920, -0.5143720371616018472, 0.000000000000000000 ) ) ;
#38421=ORIENTED_EDGE ( 'NONE', *, *, #3975, .T. ) ;
#38551=CARTESIAN_POINT ( 'NONE',  ( -110.0000000000000142, -8.000000000000000000, 9.212605237762145904 ) ) ;
#38564=CARTESIAN_POINT ( 'NONE',  ( -105.0000000000000000, 10.00000000000000000, 14.21260523776214235 ) ) ;
#38575=ORIENTED_EDGE ( 'NONE', *, *, #76180, .T. ) ;
#38625=ADVANCED_FACE ( 'NONE', ( #70143 ), #71688, .F. ) ;
#38671=CARTESIAN_POINT ( 'NONE',  ( -110.0000000000000000, 4.999999999999999112, 59.99999999999999289 ) ) ;
#38758=CARTESIAN_POINT ( 'NONE',  ( 38.90713653809340400, 79.99999999999998579, -54.99999999999999289 ) ) ;
#38759=FACE_OUTER_BOUND ( 'NONE', #32503, .T. ) ;
#38777=AXIS2_PLACEMENT_3D ( 'NONE', #42093, #96339, #3139 ) ;
#38817=EDGE_LOOP ( 'NONE', ( #18431, #39801, #77467, #46040 ) ) ;
#38993=FACE_OUTER_BOUND ( 'NONE', #56763, .T. ) ;
#39024=DIRECTION ( 'NONE',  ( 0.000000000000000000, 1.000000000000000000, -0.000000000000000000 ) ) ;
#39054=CARTESIAN_POINT ( 'NONE',  ( -19.65312891409030271, 93.06504152958497400, -54.99999999999999289 ) ) ;
#39168=CARTESIAN_POINT ( 'NONE',  ( -86.81108781737714253, 0.000000000000000000, 0.000000000000000000 ) ) ;
#39170=CARTESIAN_POINT ( 'NONE',  ( 109.9999999999999716, 10.00000000000004086, -14.21260523776213347 ) ) ;
#39179=ORIENTED_EDGE ( 'NONE', *, *, #20552, .F. ) ;
#39187=EDGE_CURVE ( 'NONE', #20674, #44016, #31393, .T. ) ;
#39204=CARTESIAN_POINT ( 'NONE',  ( 110.0000000000000142, 10.00000000000004086, 59.99999999999999289 ) ) ;
#39240=VECTOR ( 'NONE', #55961, 1000.000000000000000 ) ;
#39271=DIRECTION ( 'NONE',  ( 0.000000000000000000, 1.000000000000000000, 0.000000000000000000 ) ) ;
#39278=ORIENTED_EDGE ( 'NONE', *, *, #43091, .F. ) ;
#39339=VERTEX_POINT ( 'NONE', #40204 ) ;
#39349=LINE ( 'NONE', #9485, #22238 ) ;
#39366=FACE_OUTER_BOUND ( 'NONE', #69124, .T. ) ;
#39394=CYLINDRICAL_SURFACE ( 'NONE', #26781, 10.00000000000000355 ) ;
#39572=LINE ( 'NONE', #85770, #37199 ) ;
#39576=ADVANCED_FACE ( 'NONE', ( #85251 ), #59902, .F. ) ;
#39657=DIRECTION ( 'NONE',  ( 0.000000000000000000, 0.000000000000000000, -1.000000000000000000 ) ) ;
#39662=CARTESIAN_POINT ( 'NONE',  ( 49.80235952159635104, 79.38263285747564169, -10.00000000000000000 ) ) ;
#39689=DIRECTION ( 'NONE',  ( 1.000000000000000000, 1.156482317317871331E-15, 0.000000000000000000 ) ) ;
#39737=DIRECTION ( 'NONE',  ( 0.000000000000000000, 0.000000000000000000, 1.000000000000000000 ) ) ;
#39801=ORIENTED_EDGE ( 'NONE', *, *, #15010, .T. ) ;
#39809=CARTESIAN_POINT ( 'NONE',  ( -13.11024591527734628, 6.000000000000000000, 32.50000000000000000 ) ) ;
#39939=LINE ( 'NONE', #63265, #47941 ) ;
#39948=DIRECTION ( 'NONE',  ( -1.000000000000000000, -1.804112415015878984E-15, 0.000000000000000000 ) ) ;
#40031=CARTESIAN_POINT ( 'NONE',  ( -13.11024591527734628, 6.000000000000000000, -45.00000000000000000 ) ) ;
#40076=AXIS2_PLACEMENT_3D ( 'NONE', #8272, #62961, #33574 ) ;
#40195=AXIS2_PLACEMENT_3D ( 'NONE', #90277, #58806, #51740 ) ;
#40204=CARTESIAN_POINT ( 'NONE',  ( 110.0000000000000000, 15.00000000000000000, -9.212605237762131694 ) ) ;
#40229=AXIS2_PLACEMENT_3D ( 'NONE', #34361, #2480, #80004 ) ;
#40267=DIRECTION ( 'NONE',  ( -0.000000000000000000, -0.000000000000000000, -1.000000000000000000 ) ) ;
#40283=EDGE_CURVE ( 'NONE', #88729, #47896, #19306, .T. ) ;
#40291=ORIENTED_EDGE ( 'NONE', *, *, #27210, .F. ) ;
#40301=FACE_OUTER_BOUND ( 'NONE', #79023, .T. ) ;
#40337=DIRECTION ( 'NONE',  ( -0.000000000000000000, -0.000000000000000000, -1.000000000000000000 ) ) ;
#40358=CARTESIAN_POINT ( 'NONE',  ( -86.81108781737714253, 4.999999999999999112, -14.21260523776213347 ) ) ;
#40435=VERTEX_POINT ( 'NONE', #53919 ) ;
#40463=VECTOR ( 'NONE', #63796, 1000.000000000000000 ) ;
#40493=ORIENTED_EDGE ( 'NONE', *, *, #80291, .F. ) ;
#40587=EDGE_CURVE ( 'NONE', #82833, #57607, #93984, .T. ) ;
#40651=CARTESIAN_POINT ( 'NONE',  ( -13.11024591527723615, 6.000000000000000000, -32.50000000000017053 ) ) ;
#40702=EDGE_CURVE ( 'NONE', #35306, #2734, #48741, .T. ) ;
#40704=DIRECTION ( 'NONE',  ( 0.000000000000000000, -1.000000000000000000, 0.000000000000000000 ) ) ;
#40711=DIRECTION ( 'NONE',  ( -0.000000000000000000, -1.000000000000000000, -0.000000000000000000 ) ) ;
#40808=EDGE_LOOP ( 'NONE', ( #77204, #43660, #51150, #73637 ) ) ;
#40825=VERTEX_POINT ( 'NONE', #23507 ) ;
#40829=DIRECTION ( 'NONE',  ( 0.000000000000000000, 0.000000000000000000, 1.000000000000000000 ) ) ;
#40855=AXIS2_PLACEMENT_3D ( 'NONE', #68955, #84703, #15244 ) ;
#40888=LINE ( 'NONE', #48525, #88786 ) ;
#40913=VERTEX_POINT ( 'NONE', #30635 ) ;
#40978=PLANE ( 'NONE',  #80260 ) ;
#40980=AXIS2_PLACEMENT_3D ( 'NONE', #79962, #18127, #88086 ) ;
#41223=DIRECTION ( 'NONE',  ( -1.000000000000000000, -1.387778780781445478E-15, -0.000000000000000000 ) ) ;
#41311=EDGE_LOOP ( 'NONE', ( #79263, #8388, #22396, #66011 ) ) ;
#41316=DIRECTION ( 'NONE',  ( -1.000000000000000000, -1.804112415015878984E-15, 0.000000000000000000 ) ) ;
#41320=LINE ( 'NONE', #26644, #61087 ) ;
#41341=DIRECTION ( 'NONE',  ( 1.000000000000000000, 0.000000000000000000, -0.000000000000000000 ) ) ;
#41343=AXIS2_PLACEMENT_3D ( 'NONE', #86139, #24277, #16669 ) ;
#41379=CARTESIAN_POINT ( 'NONE',  ( -110.0000000000000000, 15.00000000000000000, 59.99999999999999289 ) ) ;
#41381=DIRECTION ( 'NONE',  ( -0.000000000000000000, -0.000000000000000000, -1.000000000000000000 ) ) ;
#41470=DIRECTION ( 'NONE',  ( -0.000000000000000000, -1.000000000000000000, -0.000000000000000000 ) ) ;
#41491=FACE_OUTER_BOUND ( 'NONE', #49852, .T. ) ;
#41495=VECTOR ( 'NONE', #52096, 1000.000000000000000 ) ;
#41553=DIRECTION ( 'NONE',  ( 1.000000000000000000, 0.000000000000000000, -1.082076799516502080E-16 ) ) ;
#41582=LINE ( 'NONE', #2613, #68975 ) ;
#41646=LINE ( 'NONE', #26964, #69455 ) ;
#41663=DIRECTION ( 'NONE',  ( -0.000000000000000000, -0.000000000000000000, -1.000000000000000000 ) ) ;
#41740=FACE_OUTER_BOUND ( 'NONE', #65857, .T. ) ;
#41817=ORIENTED_EDGE ( 'NONE', *, *, #61006, .F. ) ;
#41822=VERTEX_POINT ( 'NONE', #86468 ) ;
#41833=CARTESIAN_POINT ( 'NONE',  ( -13.11024591527734628, 27.99999999999999645, 32.50000000000000000 ) ) ;
#41834=VECTOR ( 'NONE', #83191, 1000.000000000000000 ) ;
#41851=PLANE ( 'NONE',  #6254 ) ;
#41877=CARTESIAN_POINT ( 'NONE',  ( -55.56624327025929944, 44.99999999999998579, -10.00000000000000000 ) ) ;
#41991=DIRECTION ( 'NONE',  ( 1.000000000000000000, 0.000000000000000000, 0.000000000000000000 ) ) ;
#42017=EDGE_LOOP ( 'NONE', ( #53409, #73127, #31343, #11950, #29464, #1839, #26524, #59025 ) ) ;
#42091=ORIENTED_EDGE ( 'NONE', *, *, #89789, .F. ) ;
#42093=CARTESIAN_POINT ( 'NONE',  ( -110.0000000000000142, -8.000000000000000000, 14.21260523776214590 ) ) ;
#42151=CARTESIAN_POINT ( 'NONE',  ( -105.0000000000000000, 4.999999999999999112, 59.99999999999999289 ) ) ;
#42174=LINE ( 'NONE', #52751, #97522 ) ;
#42192=VERTEX_POINT ( 'NONE', #47766 ) ;
#42195=DIRECTION ( 'NONE',  ( -1.110223024625156343E-15, 1.000000000000000000, 0.000000000000000000 ) ) ;
#42259=FACE_OUTER_BOUND ( 'NONE', #24525, .T. ) ;
#42297=DIRECTION ( 'NONE',  ( 0.000000000000000000, -1.000000000000000000, 0.000000000000000000 ) ) ;
#42384=CIRCLE ( 'NONE', #86149, 12.50000000000000000 ) ;
#42394=DIRECTION ( 'NONE',  ( 1.000000000000000000, -0.000000000000000000, -1.082076799516502080E-16 ) ) ;
#42458=EDGE_LOOP ( 'NONE', ( #98328, #55037, #57161, #76696, #69368, #10845 ) ) ;
#42488=CARTESIAN_POINT ( 'NONE',  ( -13.11024591527723437, 27.99999999999999645, -25.00000000000017053 ) ) ;
#42523=ORIENTED_EDGE ( 'NONE', *, *, #88365, .F. ) ;
#42583=VECTOR ( 'NONE', #85970, 1000.000000000000000 ) ;
#42594=FACE_OUTER_BOUND ( 'NONE', #30964, .T. ) ;
#42605=DIRECTION ( 'NONE',  ( -0.000000000000000000, 1.000000000000000000, -0.000000000000000000 ) ) ;
#42748=DIRECTION ( 'NONE',  ( -0.000000000000000000, -0.000000000000000000, -1.000000000000000000 ) ) ;
#42813=LINE ( 'NONE', #35736, #96499 ) ;
#42854=DIRECTION ( 'NONE',  ( -0.5000000000000013323, 0.8660254037844378194, 0.000000000000000000 ) ) ;
#42873=VECTOR ( 'NONE', #70179, 1000.000000000000000 ) ;
#42924=LINE ( 'NONE', #89609, #74354 ) ;
#42934=VECTOR ( 'NONE', #64869, 1000.000000000000000 ) ;
#43091=EDGE_CURVE ( 'NONE', #32489, #16870, #91236, .T. ) ;
#43128=VECTOR ( 'NONE', #91595, 1000.000000000000000 ) ;
#43152=LINE ( 'NONE', #57874, #35942 ) ;
#43192=CARTESIAN_POINT ( 'NONE',  ( 80.66987298107778770, 24.99999999999998579, 59.99999999999999289 ) ) ;
#43205=VECTOR ( 'NONE', #13556, 1000.000000000000000 ) ;
#43218=ADVANCED_FACE ( 'NONE', ( #51152 ), #28355, .T. ) ;
#43237=CARTESIAN_POINT ( 'NONE',  ( 93.96857342517718337, 15.00000000000000000, 9.212605237762133470 ) ) ;
#43333=CARTESIAN_POINT ( 'NONE',  ( 93.96857342517718337, 4.999999999999999112, -14.21260523776213347 ) ) ;
#43346=VERTEX_POINT ( 'NONE', #43932 ) ;
#43554=ADVANCED_FACE ( 'NONE', ( #74759 ), #28624, .T. ) ;
#43571=EDGE_LOOP ( 'NONE', ( #5837, #89139, #37558, #7838, #89233, #48960 ) ) ;
#43573=EDGE_CURVE ( 'NONE', #18962, #6810, #5827, .T. ) ;
#43587=ORIENTED_EDGE ( 'NONE', *, *, #91225, .F. ) ;
#43623=ORIENTED_EDGE ( 'NONE', *, *, #99221, .F. ) ;
#43660=ORIENTED_EDGE ( 'NONE', *, *, #75142, .F. ) ;
#43677=ORIENTED_EDGE ( 'NONE', *, *, #22287, .F. ) ;
#43714=DIRECTION ( 'NONE',  ( -0.000000000000000000, -0.000000000000000000, -1.000000000000000000 ) ) ;
#43743=ORIENTED_EDGE ( 'NONE', *, *, #99241, .T. ) ;
#43745=EDGE_CURVE ( 'NONE', #58927, #53652, #2347, .T. ) ;
#43783=LINE ( 'NONE', #5306, #90924 ) ;
#43798=ORIENTED_EDGE ( 'NONE', *, *, #27210, .T. ) ;
#43885=EDGE_CURVE ( 'NONE', #97093, #34316, #31649, .T. ) ;
#43924=DIRECTION ( 'NONE',  ( 0.000000000000000000, 0.000000000000000000, -1.000000000000000000 ) ) ;
#43932=CARTESIAN_POINT ( 'NONE',  ( 105.0000000000000000, 10.00000000000003197, -54.99999999999999289 ) ) ;
#43945=VERTEX_POINT ( 'NONE', #69164 ) ;
#44016=VERTEX_POINT ( 'NONE', #81680 ) ;
#44054=DIRECTION ( 'NONE',  ( 0.000000000000000000, 1.000000000000000000, 0.000000000000000000 ) ) ;
#44113=EDGE_LOOP ( 'NONE', ( #67999, #77687 ) ) ;
#44163=ORIENTED_EDGE ( 'NONE', *, *, #83384, .T. ) ;
#44178=EDGE_LOOP ( 'NONE', ( #59980, #70982 ) ) ;
#44307=ORIENTED_EDGE ( 'NONE', *, *, #11761, .F. ) ;
#44408=VERTEX_POINT ( 'NONE', #8885 ) ;
#44455=EDGE_CURVE ( 'NONE', #63624, #57758, #32181, .T. ) ;
#44458=EDGE_LOOP ( 'NONE', ( #8194, #8915, #71080, #75447 ) ) ;
#44680=EDGE_LOOP ( 'NONE', ( #60118, #50775, #6637, #88033 ) ) ;
#44750=AXIS2_PLACEMENT_3D ( 'NONE', #88627, #89137, #19688 ) ;
#44890=VECTOR ( 'NONE', #51937, 999.9999999999998863 ) ;
#44904=ORIENTED_EDGE ( 'NONE', *, *, #27524, .F. ) ;
#44997=CIRCLE ( 'NONE', #77575, 12.50000000000000000 ) ;
#45016=CIRCLE ( 'NONE', #95279, 7.500000000000000000 ) ;
#45047=CIRCLE ( 'NONE', #40195, 14.21260523776213347 ) ;
#45049=CARTESIAN_POINT ( 'NONE',  ( -13.11024591527723615, 4.999999999999999112, -32.50000000000017053 ) ) ;
#45051=CARTESIAN_POINT ( 'NONE',  ( -105.0000000000000000, 4.999999999999999112, 54.99999999999999289 ) ) ;
#45077=ORIENTED_EDGE ( 'NONE', *, *, #93770, .F. ) ;
#45104=PLANE ( 'NONE',  #2612 ) ;
#45145=VECTOR ( 'NONE', #41381, 1000.000000000000000 ) ;
#45172=CARTESIAN_POINT ( 'NONE',  ( 110.0000000000000000, 15.00000000000003908, -59.99999999999999289 ) ) ;
#45213=DIRECTION ( 'NONE',  ( -1.000000000000000000, 0.000000000000000000, 1.082076799516502204E-16 ) ) ;
#45237=CARTESIAN_POINT ( 'NONE',  ( 105.0000000000000000, 4.999999999999999112, 59.99999999999999289 ) ) ;
#45259=ORIENTED_EDGE ( 'NONE', *, *, #80889, .F. ) ;
#45399=EDGE_CURVE ( 'NONE', #37942, #61117, #230, .T. ) ;
#45552=CARTESIAN_POINT ( 'NONE',  ( -13.11024591527723615, 4.999999999999999112, -48.00000000000017053 ) ) ;
#45581=LINE ( 'NONE', #84152, #12512 ) ;
#45606=DIRECTION ( 'NONE',  ( 0.000000000000000000, 0.000000000000000000, -1.000000000000000000 ) ) ;
#45643=CARTESIAN_POINT ( 'NONE',  ( 84.99999999999998579, 14.99999999999999467, -59.99999999999999289 ) ) ;
#45694=LINE ( 'NONE', #67017, #46306 ) ;
#45753=DIRECTION ( 'NONE',  ( 1.804112415015878984E-15, -1.000000000000000000, 0.000000000000000000 ) ) ;
#45757=SHAPE_REPRESENTATION_RELATIONSHIP ( 'NONE' , 'NONE' ,  #35972, #14997 ) ;
#45773=DIRECTION ( 'NONE',  ( 0.000000000000000000, 0.000000000000000000, -1.000000000000000000 ) ) ;
#45942=ORIENTED_EDGE ( 'NONE', *, *, #83875, .F. ) ;
#46005=MANIFOLD_SOLID_BREP ( 'Move Face1', #89593 ) ;
#46020=DIRECTION ( 'NONE',  ( -0.000000000000000000, -1.000000000000000000, -0.000000000000000000 ) ) ;
#46040=ORIENTED_EDGE ( 'NONE', *, *, #65026, .F. ) ;
#46042=CARTESIAN_POINT ( 'NONE',  ( 51.80235952159637236, 80.00000000000000000, 59.99999999999999289 ) ) ;
#46063=DIRECTION ( 'NONE',  ( -0.5000000000000014433, 0.8660254037844379305, 0.000000000000000000 ) ) ;
#46065=EDGE_CURVE ( 'NONE', #64385, #40435, #62266, .T. ) ;
#46100=CARTESIAN_POINT ( 'NONE',  ( 26.11609497015385983, 119.4899152597536869, 54.99999999999999289 ) ) ;
#46129=PRODUCT_CONTEXT ( 'NONE', #67032, 'mechanical' ) ;
#46136=DIRECTION ( 'NONE',  ( -0.000000000000000000, -1.000000000000000000, -0.000000000000000000 ) ) ;
#46213=CARTESIAN_POINT ( 'NONE',  ( 48.91560817564824504, 80.00000000000000000, 10.00000000000000178 ) ) ;
#46224=VECTOR ( 'NONE', #51059, 1000.000000000000114 ) ;
#46263=EDGE_CURVE ( 'NONE', #9173, #58927, #50087, .T. ) ;
#46306=VECTOR ( 'NONE', #43714, 1000.000000000000000 ) ;
#46366=CYLINDRICAL_SURFACE ( 'NONE', #64628, 10.00000000000000355 ) ;
#46406=VECTOR ( 'NONE', #7350, 1000.000000000000000 ) ;
#46420=LINE ( 'NONE', #79389, #62578 ) ;
#46453=ORIENTED_EDGE ( 'NONE', *, *, #58740, .F. ) ;
#46570=EDGE_CURVE ( 'NONE', #43346, #40913, #830, .T. ) ;
#46573=LINE ( 'NONE', #23781, #30230 ) ;
#46592=DIRECTION ( 'NONE',  ( 0.000000000000000000, 0.000000000000000000, 1.000000000000000000 ) ) ;
#46607=VECTOR ( 'NONE', #45773, 1000.000000000000000 ) ;
#46654=EDGE_CURVE ( 'NONE', #28403, #43346, #67889, .T. ) ;
#46691=CIRCLE ( 'NONE', #6269, 10.00000000000001066 ) ;
#46710=CARTESIAN_POINT ( 'NONE',  ( -86.81108781737714253, 15.00000000000000000, 9.212605237762131694 ) ) ;
#46727=ORIENTED_EDGE ( 'NONE', *, *, #40587, .T. ) ;
#46740=ORIENTED_EDGE ( 'NONE', *, *, #10312, .F. ) ;
#46744=CARTESIAN_POINT ( 'NONE',  ( 84.99999999999998579, 14.99999999999999467, 59.99999999999999289 ) ) ;
#46746=AXIS2_PLACEMENT_3D ( 'NONE', #13110, #60657, #67789 ) ;
#46795=CARTESIAN_POINT ( 'NONE',  ( 79.99999999999998579, 9.999999999999985789, 59.99999999999999289 ) ) ;
#46965=VECTOR ( 'NONE', #49002, 1000.000000000000000 ) ;
#47021=CARTESIAN_POINT ( 'NONE',  ( -13.11024591527723615, 4.999999999999999112, -32.50000000000017053 ) ) ;
#47080=CARTESIAN_POINT ( 'NONE',  ( -110.0000000000000000, 0.000000000000000000, -59.99999999999999289 ) ) ;
#47140=FACE_OUTER_BOUND ( 'NONE', #73508, .T. ) ;
#47144=EDGE_CURVE ( 'NONE', #40913, #6085, #35095, .T. ) ;
#47152=DIRECTION ( 'NONE',  ( 1.000000000000000000, 0.000000000000000000, -5.984665299743594308E-16 ) ) ;
#47165=CYLINDRICAL_SURFACE ( 'NONE', #9546, 15.50000000000000000 ) ;
#47193=DIRECTION ( 'NONE',  ( 0.2237140788069379993, 0.9746548163034761680, 0.000000000000000000 ) ) ;
#47272=EDGE_CURVE ( 'NONE', #33261, #77716, #21884, .T. ) ;
#47289=FACE_OUTER_BOUND ( 'NONE', #84848, .T. ) ;
#47315=DIRECTION ( 'NONE',  ( 1.156482317317871331E-15, -1.000000000000000000, 0.000000000000000000 ) ) ;
#47345=UNCERTAINTY_MEASURE_WITH_UNIT (LENGTH_MEASURE( 1.000000000000000082E-05 ), #60965, 'distance_accuracy_value', 'NONE');
#47360=CARTESIAN_POINT ( 'NONE',  ( -86.81108781737714253, -8.000000000000000000, 0.000000000000000000 ) ) ;
#47369=DIRECTION ( 'NONE',  ( 1.000000000000000000, 0.000000000000000000, -5.984665299743594308E-16 ) ) ;
#47426=EDGE_LOOP ( 'NONE', ( #62411, #20796 ) ) ;
#47433=CYLINDRICAL_SURFACE ( 'NONE', #64698, 12.50000000000000000 ) ;
#47470=EDGE_CURVE ( 'NONE', #42192, #80375, #59246, .T. ) ;
#47535=CARTESIAN_POINT ( 'NONE',  ( -13.11024591527723615, 15.00000000000000000, -40.00000000000016342 ) ) ;
#47538=VERTEX_POINT ( 'NONE', #98295 ) ;
#47667=ORIENTED_EDGE ( 'NONE', *, *, #80380, .F. ) ;
#47763=ADVANCED_FACE ( 'NONE', ( #64759 ), #80495, .F. ) ;
#47766=CARTESIAN_POINT ( 'NONE',  ( -105.0000000000000000, 4.999999999999999112, 14.21260523776214235 ) ) ;
#47786=CARTESIAN_POINT ( 'NONE',  ( 93.96857342517718337, -8.000000000000000000, 14.21260523776213347 ) ) ;
#47797=ORIENTED_EDGE ( 'NONE', *, *, #355, .T. ) ;
#47811=DIRECTION ( 'NONE',  ( 1.000000000000000000, 1.804112415015878984E-15, 0.000000000000000000 ) ) ;
#47828=AXIS2_PLACEMENT_3D ( 'NONE', #46042, #7558, #76976 ) ;
#47853=DIRECTION ( 'NONE',  ( 1.000000000000000000, 0.000000000000000000, -0.000000000000000000 ) ) ;
#47876=DIRECTION ( 'NONE',  ( 0.000000000000000000, 0.000000000000000000, 1.000000000000000000 ) ) ;
#47896=VERTEX_POINT ( 'NONE', #83473 ) ;
#47902=CYLINDRICAL_SURFACE ( 'NONE', #33501, 14.21260523776213347 ) ;
#47916=DIRECTION ( 'NONE',  ( -0.5000000000000011102, -0.8660254037844380415, -0.000000000000000000 ) ) ;
#47917=CARTESIAN_POINT ( 'NONE',  ( -19.65312891409015350, 9.999999999999801048, -54.99999999999999289 ) ) ;
#47941=VECTOR ( 'NONE', #49560, 1000.000000000000114 ) ;
#48016=CYLINDRICAL_SURFACE ( 'NONE', #6809, 15.50000000000000000 ) ;
#48017=ADVANCED_FACE ( 'NONE', ( #93559 ), #63123, .F. ) ;
#48095=AXIS2_PLACEMENT_3D ( 'NONE', #52732, #83695, #68439 ) ;
#48101=EDGE_LOOP ( 'NONE', ( #61807, #48546, #22777, #707 ) ) ;
#48107=ADVANCED_FACE ( 'NONE', ( #24712 ), #39394, .F. ) ;
#48150=CARTESIAN_POINT ( 'NONE',  ( -19.65312891409030271, 93.06504152958497400, 59.99999999999999289 ) ) ;
#48169=VERTEX_POINT ( 'NONE', #91000 ) ;
#48176=DIRECTION ( 'NONE',  ( 0.000000000000000000, 0.000000000000000000, -1.000000000000000000 ) ) ;
#48199=LINE ( 'NONE', #79146, #43128 ) ;
#48243=VECTOR ( 'NONE', #84289, 1000.000000000000000 ) ;
#48285=CARTESIAN_POINT ( 'NONE',  ( -110.0000000000000000, 15.00000000000000000, 59.99999999999999289 ) ) ;
#48422=AXIS2_PLACEMENT_3D ( 'NONE', #12313, #7554, #15645 ) ;
#48454=ORIENTED_EDGE ( 'NONE', *, *, #16743, .F. ) ;
#48468=VERTEX_POINT ( 'NONE', #31510 ) ;
#48525=CARTESIAN_POINT ( 'NONE',  ( -105.0000000000000000, 0.000000000000000000, -14.21260523776211215 ) ) ;
#48546=ORIENTED_EDGE ( 'NONE', *, *, #8589, .F. ) ;
#48549=CARTESIAN_POINT ( 'NONE',  ( 110.0000000000000000, 0.000000000000000000, -59.99999999999999289 ) ) ;
#48622=ADVANCED_FACE ( 'NONE', ( #41491 ), #40978, .F. ) ;
#48673=ORIENTED_EDGE ( 'NONE', *, *, #47144, .T. ) ;
#48710=ORIENTED_EDGE ( 'NONE', *, *, #24538, .T. ) ;
#48741=LINE ( 'NONE', #79171, #100133 ) ;
#48755=DIRECTION ( 'NONE',  ( 0.000000000000000000, 0.000000000000000000, 1.000000000000000000 ) ) ;
#48788=DIRECTION ( 'NONE',  ( 0.000000000000000000, 0.000000000000000000, 1.000000000000000000 ) ) ;
#48939=VERTEX_POINT ( 'NONE', #32657 ) ;
#48960=ORIENTED_EDGE ( 'NONE', *, *, #59559, .T. ) ;
#48966=PLANE ( 'NONE',  #5991 ) ;
#49002=DIRECTION ( 'NONE',  ( -0.000000000000000000, -0.000000000000000000, -1.000000000000000000 ) ) ;
#49004=DIRECTION ( 'NONE',  ( -0.000000000000000000, 1.000000000000000000, -0.000000000000000000 ) ) ;
#49025=ORIENTED_EDGE ( 'NONE', *, *, #71457, .F. ) ;
#49027=LINE ( 'NONE', #35684, #85350 ) ;
#49103=LINE ( 'NONE', #78012, #40463 ) ;
#49158=VERTEX_POINT ( 'NONE', #21942 ) ;
#49173=EDGE_CURVE ( 'NONE', #16631, #35859, #75660, .T. ) ;
#49213=EDGE_LOOP ( 'NONE', ( #59418, #82569, #85994, #6596, #80340, #83853, #54476, #21965 ) ) ;
#49297=VERTEX_POINT ( 'NONE', #16834 ) ;
#49329=DIRECTION ( 'NONE',  ( -0.000000000000000000, -1.000000000000000000, -0.000000000000000000 ) ) ;
#49340=CARTESIAN_POINT ( 'NONE',  ( -55.56624327025929944, 44.99999999999998579, -59.99999999999999289 ) ) ;
#49412=VERTEX_POINT ( 'NONE', #34534 ) ;
#49452=CARTESIAN_POINT ( 'NONE',  ( -19.65312891409030271, 93.06504152958497400, 10.00000000000000000 ) ) ;
#49508=DIRECTION ( 'NONE',  ( 0.000000000000000000, 1.000000000000000000, 0.000000000000000000 ) ) ;
#49525=VERTEX_POINT ( 'NONE', #78537 ) ;
#49560=DIRECTION ( 'NONE',  ( -0.5000000000000011102, -0.8660254037844380415, 0.000000000000000000 ) ) ;
#49580=DIRECTION ( 'NONE',  ( -1.000000000000000000, 0.000000000000000000, 1.082076799516502080E-16 ) ) ;
#49587=CARTESIAN_POINT ( 'NONE',  ( -13.11024591527734451, 6.000000000000000000, -20.00000000000000000 ) ) ;
#49612=CIRCLE ( 'NONE', #44750, 9.212605237762131694 ) ;
#49649=CIRCLE ( 'NONE', #31853, 7.499999999999996447 ) ;
#49654=ORIENTED_EDGE ( 'NONE', *, *, #93833, .T. ) ;
#49793=FACE_OUTER_BOUND ( 'NONE', #48101, .T. ) ;
#49852=EDGE_LOOP ( 'NONE', ( #17758, #38041 ) ) ;
#49876=DIRECTION ( 'NONE',  ( 0.000000000000000000, -0.000000000000000000, -1.000000000000000000 ) ) ;
#49979=ORIENTED_EDGE ( 'NONE', *, *, #80889, .T. ) ;
#49994=LINE ( 'NONE', #96137, #58710 ) ;
#49995=DIRECTION ( 'NONE',  ( 1.000000000000000000, 0.000000000000000000, -5.984665299743594308E-16 ) ) ;
#50057=DIRECTION ( 'NONE',  ( -1.110223024625156343E-15, 1.000000000000000000, 0.000000000000000000 ) ) ;
#50087=LINE ( 'NONE', #81044, #57424 ) ;
#50179=ORIENTED_EDGE ( 'NONE', *, *, #90752, .F. ) ;
#50191=ORIENTED_EDGE ( 'NONE', *, *, #89062, .F. ) ;
#50360=EDGE_CURVE ( 'NONE', #22518, #89960, #21345, .T. ) ;
#50489=CARTESIAN_POINT ( 'NONE',  ( -110.0000000000000000, 0.000000000000000000, 59.99999999999999289 ) ) ;
#50517=VERTEX_POINT ( 'NONE', #45552 ) ;
#50546=EDGE_CURVE ( 'NONE', #75741, #6085, #100284, .T. ) ;
#50576=ORIENTED_EDGE ( 'NONE', *, *, #18904, .T. ) ;
#50608=AXIS2_PLACEMENT_3D ( 'NONE', #19523, #33191, #26101 ) ;
#50626=ORIENTED_EDGE ( 'NONE', *, *, #18191, .F. ) ;
#50646=ORIENTED_EDGE ( 'NONE', *, *, #61006, .T. ) ;
#50687=EDGE_CURVE ( 'NONE', #97333, #49525, #39939, .T. ) ;
#50704=VECTOR ( 'NONE', #47369, 1000.000000000000000 ) ;
#50710=CARTESIAN_POINT ( 'NONE',  ( 51.80235952159636525, 85.00000000000000000, -59.99999999999999289 ) ) ;
#50742=EDGE_CURVE ( 'NONE', #91371, #61436, #49612, .T. ) ;
#50754=CARTESIAN_POINT ( 'NONE',  ( -70.00000000000000000, 20.00000000000000000, 59.99999999999999289 ) ) ;
#50775=ORIENTED_EDGE ( 'NONE', *, *, #16743, .T. ) ;
#50797=CARTESIAN_POINT ( 'NONE',  ( 49.80235952159635815, 85.00000000000000000, -10.00000000000000000 ) ) ;
#50840=ORIENTED_EDGE ( 'NONE', *, *, #43745, .F. ) ;
#50846=VECTOR ( 'NONE', #22575, 1000.000000000000000 ) ;
#51059=DIRECTION ( 'NONE',  ( -0.5000000000000011102, -0.8660254037844380415, 0.000000000000000000 ) ) ;
#51120=ADVANCED_FACE ( 'NONE', ( #88853 ), #73592, .F. ) ;
#51150=ORIENTED_EDGE ( 'NONE', *, *, #49173, .F. ) ;
#51152=FACE_OUTER_BOUND ( 'NONE', #12680, .T. ) ;
#51287=EDGE_LOOP ( 'NONE', ( #71757, #15381, #17372, #66318 ) ) ;
#51338=DIRECTION ( 'NONE',  ( -0.000000000000000000, -1.000000000000000000, -0.000000000000000000 ) ) ;
#51404=PLANE ( 'NONE',  #72612 ) ;
#51473=DIRECTION ( 'NONE',  ( -0.000000000000000000, -1.000000000000000000, -0.000000000000000000 ) ) ;
#51569=PLANE ( 'NONE',  #64150 ) ;
#51576=ADVANCED_FACE ( 'NONE', ( #34225 ), #47902, .T. ) ;
#51588=ADVANCED_FACE ( 'NONE', ( #40301 ), #11936, .T. ) ;
#51622=VECTOR ( 'NONE', #74828, 999.9999999999998863 ) ;
#51648=PLANE ( 'NONE',  #56362 ) ;
#51664=CARTESIAN_POINT ( 'NONE',  ( -51.42721978966704910, 42.16899896210639298, 54.99999999999999289 ) ) ;
#51699=VECTOR ( 'NONE', #14485, 1000.000000000000000 ) ;
#51740=DIRECTION ( 'NONE',  ( 1.000000000000000000, 1.830829162166278276E-15, 0.000000000000000000 ) ) ;
#51773=DIRECTION ( 'NONE',  ( -0.4999999999999997780, -0.8660254037844387076, 0.000000000000000000 ) ) ;
#51782=VERTEX_POINT ( 'NONE', #11698 ) ;
#51841=CIRCLE ( 'NONE', #98783, 14.21260523776213347 ) ;
#51867=EDGE_CURVE ( 'NONE', #31869, #50517, #78579, .T. ) ;
#51900=DIRECTION ( 'NONE',  ( 0.000000000000000000, 0.000000000000000000, -1.000000000000000000 ) ) ;
#51937=DIRECTION ( 'NONE',  ( -0.5000000000000014433, 0.8660254037844379305, 0.000000000000000000 ) ) ;
#52069=ORIENTED_EDGE ( 'NONE', *, *, #4573, .F. ) ;
#52082=DIRECTION ( 'NONE',  ( 1.000000000000000000, 0.000000000000000000, -0.000000000000000000 ) ) ;
#52090=CARTESIAN_POINT ( 'NONE',  ( -13.11024591527723615, 27.99999999999999645, -32.50000000000017053 ) ) ;
#52096=DIRECTION ( 'NONE',  ( 0.000000000000000000, 0.000000000000000000, -1.000000000000000000 ) ) ;
#52221=VECTOR ( 'NONE', #30588, 1000.000000000000000 ) ;
#52278=DIRECTION ( 'NONE',  ( 0.000000000000000000, 0.000000000000000000, -1.000000000000000000 ) ) ;
#52325=EDGE_CURVE ( 'NONE', #44408, #47896, #28070, .T. ) ;
#52387=LINE ( 'NONE', #61960, #26347 ) ;
#52410=ORIENTED_EDGE ( 'NONE', *, *, #35652, .F. ) ;
#52455=VERTEX_POINT ( 'NONE', #7659 ) ;
#52657=CARTESIAN_POINT ( 'NONE',  ( -13.11024591527734451, 6.000000000000000000, 45.00000000000000000 ) ) ;
#52732=CARTESIAN_POINT ( 'NONE',  ( 110.0000000000000000, 0.000000000000000000, 59.99999999999999289 ) ) ;
#52751=CARTESIAN_POINT ( 'NONE',  ( 79.99999999999998579, 9.999999999999985789, 2.622423327744133559 ) ) ;
#52782=ORIENTED_EDGE ( 'NONE', *, *, #95988, .T. ) ;
#52819=CARTESIAN_POINT ( 'NONE',  ( -65.66987298107781612, 17.49999999999999645, -10.00000000000000178 ) ) ;
#52976=LINE ( 'NONE', #100097, #35154 ) ;
#52982=CARTESIAN_POINT ( 'NONE',  ( -65.00000000000000000, 93.06504152958497400, 54.99999999999999289 ) ) ;
#52993=LINE ( 'NONE', #7906, #37410 ) ;
#53003=VERTEX_POINT ( 'NONE', #74305 ) ;
#53077=EDGE_CURVE ( 'NONE', #8604, #40825, #76753, .T. ) ;
#53194=ORIENTED_EDGE ( 'NONE', *, *, #83832, .F. ) ;
#53281=ORIENTED_EDGE ( 'NONE', *, *, #71482, .F. ) ;
#53323=DIRECTION ( 'NONE',  ( -0.000000000000000000, -0.000000000000000000, -1.000000000000000000 ) ) ;
#53347=VECTOR ( 'NONE', #49995, 1000.000000000000000 ) ;
#53394=CARTESIAN_POINT ( 'NONE',  ( -55.56624327025929944, 44.99999999999998579, 59.99999999999999289 ) ) ;
#53409=ORIENTED_EDGE ( 'NONE', *, *, #98872, .F. ) ;
#53415=DIRECTION ( 'NONE',  ( -0.000000000000000000, -0.000000000000000000, -1.000000000000000000 ) ) ;
#53530=DIRECTION ( 'NONE',  ( -0.000000000000000000, 0.000000000000000000, -1.000000000000000000 ) ) ;
#53538=ORIENTED_EDGE ( 'NONE', *, *, #98732, .F. ) ;
#53572=CARTESIAN_POINT ( 'NONE',  ( -13.11024591527734628, 27.99999999999999645, 17.00000000000000000 ) ) ;
#53652=VERTEX_POINT ( 'NONE', #69529 ) ;
#53665=ORIENTED_EDGE ( 'NONE', *, *, #37494, .T. ) ;
#53706=ORIENTED_EDGE ( 'NONE', *, *, #67829, .F. ) ;
#53740=FACE_OUTER_BOUND ( 'NONE', #98417, .T. ) ;
#53773=ORIENTED_EDGE ( 'NONE', *, *, #80291, .T. ) ;
#53782=AXIS2_PLACEMENT_3D ( 'NONE', #69773, #380, #66906 ) ;
#53819=DIRECTION ( 'NONE',  ( 0.000000000000000000, 0.000000000000000000, -1.000000000000000000 ) ) ;
#53850=PLANE ( 'NONE',  #27988 ) ;
#53919=CARTESIAN_POINT ( 'NONE',  ( 84.99999999999997158, 27.49999999999999645, -59.99999999999999289 ) ) ;
#54085=DIRECTION ( 'NONE',  ( -0.000000000000000000, 1.000000000000000000, -0.000000000000000000 ) ) ;
#54144=ORIENTED_EDGE ( 'NONE', *, *, #88067, .F. ) ;
#54245=FACE_OUTER_BOUND ( 'NONE', #22739, .T. ) ;
#54247=ORIENTED_EDGE ( 'NONE', *, *, #79915, .F. ) ;
#54252=AXIS2_PLACEMENT_3D ( 'NONE', #3521, #26308, #11124 ) ;
#54323=AXIS2_PLACEMENT_3D ( 'NONE', #83274, #51338, #13842 ) ;
#54350=FACE_BOUND ( 'NONE', #67617, .T. ) ;
#54363=ORIENTED_EDGE ( 'NONE', *, *, #55295, .F. ) ;
#54378=EDGE_LOOP ( 'NONE', ( #53665, #70991 ) ) ;
#54472=CARTESIAN_POINT ( 'NONE',  ( 39.80235952159635815, 84.99999999999998579, 10.00000000000000000 ) ) ;
#54476=ORIENTED_EDGE ( 'NONE', *, *, #4573, .T. ) ;
#54554=CIRCLE ( 'NONE', #99852, 9.212605237762131694 ) ;
#54631=VECTOR ( 'NONE', #61184, 1000.000000000000000 ) ;
#54639=EDGE_CURVE ( 'NONE', #76018, #53003, #41582, .T. ) ;
#54641=VECTOR ( 'NONE', #12804, 1000.000000000000000 ) ;
#54664=DIRECTION ( 'NONE',  ( 0.000000000000000000, 0.000000000000000000, 1.000000000000000000 ) ) ;
#54668=DIRECTION ( 'NONE',  ( -0.000000000000000000, -0.000000000000000000, -1.000000000000000000 ) ) ;
#54679=CIRCLE ( 'NONE', #1350, 10.00000000000001066 ) ;
#54703=VERTEX_POINT ( 'NONE', #36474 ) ;
#54741=CYLINDRICAL_SURFACE ( 'NONE', #86135, 7.500000000000000000 ) ;
#54763=AXIS2_PLACEMENT_3D ( 'NONE', #95214, #32857, #26271 ) ;
#54781=FACE_OUTER_BOUND ( 'NONE', #56381, .T. ) ;
#54864=DIRECTION ( 'NONE',  ( -0.000000000000000000, 1.000000000000000000, -0.000000000000000000 ) ) ;
#54882=ADVANCED_FACE ( 'NONE', ( #20681 ), #51569, .T. ) ;
#54899=ORIENTED_EDGE ( 'NONE', *, *, #94761, .F. ) ;
#54930=AXIS2_PLACEMENT_3D ( 'NONE', #73715, #46136, #3816 ) ;
#54931=ORIENTED_EDGE ( 'NONE', *, *, #33555, .F. ) ;
#55005=CARTESIAN_POINT ( 'NONE',  ( -110.0000000000000000, 15.00000000000000000, -59.99999999999999289 ) ) ;
#55013=DIRECTION ( 'NONE',  ( -0.000000000000000000, -1.000000000000000000, -0.000000000000000000 ) ) ;
#55037=ORIENTED_EDGE ( 'NONE', *, *, #19017, .T. ) ;
#55109=FACE_OUTER_BOUND ( 'NONE', #81743, .T. ) ;
#55118=EDGE_LOOP ( 'NONE', ( #61648, #50646, #89354, #77255 ) ) ;
#55162=ORIENTED_EDGE ( 'NONE', *, *, #93233, .T. ) ;
#55170=CARTESIAN_POINT ( 'NONE',  ( 84.99999999999997158, 27.49999999999999645, 59.99999999999999289 ) ) ;
#55201=LINE ( 'NONE', #61312, #16089 ) ;
#55295=EDGE_CURVE ( 'NONE', #9320, #76847, #67512, .T. ) ;
#55325=CARTESIAN_POINT ( 'NONE',  ( 79.99999999999998579, 9.999999999999985789, 54.99999999999999289 ) ) ;
#55389=ORIENTED_EDGE ( 'NONE', *, *, #76724, .T. ) ;
#55405=DIRECTION ( 'NONE',  ( 1.804112415015878984E-15, -1.000000000000000000, 0.000000000000000000 ) ) ;
#55416=DIRECTION ( 'NONE',  ( 0.000000000000000000, -1.000000000000000000, 0.000000000000000000 ) ) ;
#55445=DIRECTION ( 'NONE',  ( -0.000000000000000000, 1.000000000000000000, -0.000000000000000000 ) ) ;
#55531=EDGE_CURVE ( 'NONE', #10673, #49297, #97824, .T. ) ;
#55534=CARTESIAN_POINT ( 'NONE',  ( -19.65312891409028850, 79.99999999999991473, -54.99999999999999289 ) ) ;
#55595=DIRECTION ( 'NONE',  ( 0.8660254037844378194, 0.5000000000000015543, -0.000000000000000000 ) ) ;
#55597=DIRECTION ( 'NONE',  ( 0.000000000000000000, 1.000000000000000000, 0.000000000000000000 ) ) ;
#55607=ORIENTED_EDGE ( 'NONE', *, *, #59099, .F. ) ;
#55618=LINE ( 'NONE', #48549, #75745 ) ;
#55656=EDGE_CURVE ( 'NONE', #40825, #14428, #46573, .T. ) ;
#55657=ORIENTED_EDGE ( 'NONE', *, *, #30852, .F. ) ;
#55670=CARTESIAN_POINT ( 'NONE',  ( 93.96857342517719758, 10.00000000000001243, 0.000000000000000000 ) ) ;
#55761=DIRECTION ( 'NONE',  ( 1.000000000000000000, 0.000000000000000000, -0.000000000000000000 ) ) ;
#55924=VERTEX_POINT ( 'NONE', #74133 ) ;
#55928=AXIS2_PLACEMENT_3D ( 'NONE', #714, #53415, #93963 ) ;
#55961=DIRECTION ( 'NONE',  ( -0.000000000000000000, -0.000000000000000000, -1.000000000000000000 ) ) ;
#56015=DIRECTION ( 'NONE',  ( -0.000000000000000000, -1.000000000000000000, -0.000000000000000000 ) ) ;
#56064=DIRECTION ( 'NONE',  ( -0.8660254037844379305, -0.5000000000000014433, 0.000000000000000000 ) ) ;
#56092=FACE_OUTER_BOUND ( 'NONE', #77106, .T. ) ;
#56174=CARTESIAN_POINT ( 'NONE',  ( 84.99999999999998579, 14.99999999999999467, -2.106367960268910711 ) ) ;
#56278=PLANE ( 'NONE',  #32076 ) ;
#56355=DIRECTION ( 'NONE',  ( 0.000000000000000000, -1.000000000000000000, 0.000000000000000000 ) ) ;
#56362=AXIS2_PLACEMENT_3D ( 'NONE', #75970, #60212, #98258 ) ;
#56368=CIRCLE ( 'NONE', #54763, 60.00000000000001421 ) ;
#56381=EDGE_LOOP ( 'NONE', ( #93181, #66278, #76522, #6682 ) ) ;
#56445=AXIS2_PLACEMENT_3D ( 'NONE', #35004, #3152, #27429 ) ;
#56451=EDGE_LOOP ( 'NONE', ( #16447, #4359, #30233, #1120 ) ) ;
#56503=ORIENTED_EDGE ( 'NONE', *, *, #40702, .F. ) ;
#56512=AXIS2_PLACEMENT_3D ( 'NONE', #17889, #54864, #48788 ) ;
#56629=EDGE_LOOP ( 'NONE', ( #37928, #35512, #90623, #1481 ) ) ;
#56656=CIRCLE ( 'NONE', #13009, 9.212605237762131694 ) ;
#56705=EDGE_LOOP ( 'NONE', ( #91835, #33839, #6415, #10043 ) ) ;
#56719=ORIENTED_EDGE ( 'NONE', *, *, #80380, .T. ) ;
#56763=EDGE_LOOP ( 'NONE', ( #5970, #97763, #53194, #9384 ) ) ;
#56883=ORIENTED_EDGE ( 'NONE', *, *, #14525, .F. ) ;
#57003=CARTESIAN_POINT ( 'NONE',  ( 110.0000000000000000, -8.000000000000000000, -9.212605237762131694 ) ) ;
#57079=DIRECTION ( 'NONE',  ( 0.000000000000000000, 0.000000000000000000, 1.000000000000000000 ) ) ;
#57140=CARTESIAN_POINT ( 'NONE',  ( -13.11024591527734628, 0.000000000000000000, -32.50000000000000000 ) ) ;
#57146=AXIS2_PLACEMENT_3D ( 'NONE', #36181, #97047, #51900 ) ;
#57149=ORIENTED_EDGE ( 'NONE', *, *, #100044, .F. ) ;
#57161=ORIENTED_EDGE ( 'NONE', *, *, #67829, .T. ) ;
#57163=VERTEX_POINT ( 'NONE', #32393 ) ;
#57171=DIRECTION ( 'NONE',  ( -1.082076799516502080E-16, 0.000000000000000000, -1.000000000000000000 ) ) ;
#57289=PLANE ( 'NONE',  #38777 ) ;
#57332=ADVANCED_FACE ( 'NONE', ( #91609, #62658 ), #92615, .T. ) ;
#57370=CARTESIAN_POINT ( 'NONE',  ( 105.0000000000000142, 93.06504152958497400, -54.99999999999999289 ) ) ;
#57399=EDGE_LOOP ( 'NONE', ( #88104, #56719, #97689, #66472 ) ) ;
#57418=VERTEX_POINT ( 'NONE', #77722 ) ;
#57424=VECTOR ( 'NONE', #41470, 1000.000000000000000 ) ;
#57434=VECTOR ( 'NONE', #79271, 1000.000000000000000 ) ;
#57436=DIRECTION ( 'NONE',  ( -0.000000000000000000, -1.000000000000000000, -0.000000000000000000 ) ) ;
#57461=PLANE ( 'NONE',  #32835 ) ;
#57562=ORIENTED_EDGE ( 'NONE', *, *, #29469, .F. ) ;
#57607=VERTEX_POINT ( 'NONE', #45051 ) ;
#57615=ORIENTED_EDGE ( 'NONE', *, *, #35325, .T. ) ;
#57642=CARTESIAN_POINT ( 'NONE',  ( 79.99999999999990052, 93.06504152958508769, 54.99999999999999289 ) ) ;
#57758=VERTEX_POINT ( 'NONE', #20169 ) ;
#57777=DIRECTION ( 'NONE',  ( 0.000000000000000000, 1.000000000000000000, -0.000000000000000000 ) ) ;
#57818=EDGE_CURVE ( 'NONE', #2619, #79527, #18979, .T. ) ;
#57860=ADVANCED_FACE ( 'NONE', ( #91086 ), #82987, .T. ) ;
#57874=CARTESIAN_POINT ( 'NONE',  ( -110.0000000000000000, 0.000000000000000000, -59.99999999999999289 ) ) ;
#57959=ORIENTED_EDGE ( 'NONE', *, *, #91160, .T. ) ;
#57968=CARTESIAN_POINT ( 'NONE',  ( -19.65312891409030271, 93.06504152958497400, 54.99999999999999289 ) ) ;
#57977=DIRECTION ( 'NONE',  ( -0.000000000000000000, -1.000000000000000000, -0.000000000000000000 ) ) ;
#57979=CARTESIAN_POINT ( 'NONE',  ( -62.06645187246645889, 33.74130844118090522, 10.00000000000000000 ) ) ;
#57986=FACE_OUTER_BOUND ( 'NONE', #6355, .T. ) ;
#58018=CIRCLE ( 'NONE', #14340, 7.500000000000000000 ) ;
#58019=CARTESIAN_POINT ( 'NONE',  ( 105.0000000000000000, 10.00000000000003197, -14.21260523776213347 ) ) ;
#58073=VERTEX_POINT ( 'NONE', #96586 ) ;
#58080=EDGE_CURVE ( 'NONE', #9320, #49412, #75746, .T. ) ;
#58082=CARTESIAN_POINT ( 'NONE',  ( 70.48286763772495078, 52.64441083166268243, 0.000000000000000000 ) ) ;
#58113=DIRECTION ( 'NONE',  ( 0.000000000000000000, 1.000000000000000000, 0.000000000000000000 ) ) ;
#58159=ORIENTED_EDGE ( 'NONE', *, *, #46654, .F. ) ;
#58200=VECTOR ( 'NONE', #39657, 1000.000000000000000 ) ;
#58253=CARTESIAN_POINT ( 'NONE',  ( 105.0000000000000000, 10.00000000000003197, 54.99999999999999289 ) ) ;
#58271=LINE ( 'NONE', #95837, #10758 ) ;
#58327=ORIENTED_EDGE ( 'NONE', *, *, #23207, .T. ) ;
#58345=CARTESIAN_POINT ( 'NONE',  ( -13.11024591527734628, 0.000000000000000000, -45.00000000000000000 ) ) ;
#58367=EDGE_CURVE ( 'NONE', #49412, #12543, #41320, .T. ) ;
#58501=DIRECTION ( 'NONE',  ( -1.000000000000000000, 0.000000000000000000, 5.984665299743594308E-16 ) ) ;
#58513=ORIENTED_EDGE ( 'NONE', *, *, #91160, .F. ) ;
#58609=EDGE_LOOP ( 'NONE', ( #82638, #5942 ) ) ;
#58658=CIRCLE ( 'NONE', #14978, 15.50000000000000000 ) ;
#58699=VECTOR ( 'NONE', #78942, 1000.000000000000000 ) ;
#58710=VECTOR ( 'NONE', #4903, 1000.000000000000114 ) ;
#58715=ORIENTED_EDGE ( 'NONE', *, *, #39187, .T. ) ;
#58740=EDGE_CURVE ( 'NONE', #61222, #69960, #77987, .T. ) ;
#58741=VERTEX_POINT ( 'NONE', #1982 ) ;
#58806=DIRECTION ( 'NONE',  ( -1.804112415015878984E-15, 1.000000000000000000, -0.000000000000000000 ) ) ;
#58807=CARTESIAN_POINT ( 'NONE',  ( 49.65150239490934325, 78.72539382324356438, 59.99999999999999289 ) ) ;
#58927=VERTEX_POINT ( 'NONE', #90105 ) ;
#59025=ORIENTED_EDGE ( 'NONE', *, *, #24976, .F. ) ;
#59092=EDGE_CURVE ( 'NONE', #36246, #31869, #5910, .T. ) ;
#59099=EDGE_CURVE ( 'NONE', #36590, #32767, #32249, .T. ) ;
#59131=VECTOR ( 'NONE', #57977, 1000.000000000000000 ) ;
#59204=EDGE_LOOP ( 'NONE', ( #85256, #13040, #3355, #40493 ) ) ;
#59232=CARTESIAN_POINT ( 'NONE',  ( -110.0000000000000000, 10.00000000000000000, 59.99999999999999289 ) ) ;
#59246=LINE ( 'NONE', #22268, #96374 ) ;
#59332=LINE ( 'NONE', #90312, #28291 ) ;
#59406=VECTOR ( 'NONE', #76031, 1000.000000000000000 ) ;
#59418=ORIENTED_EDGE ( 'NONE', *, *, #47144, .F. ) ;
#59471=DIRECTION ( 'NONE',  ( -1.110223024625156343E-15, 1.000000000000000000, 0.000000000000000000 ) ) ;
#59517=ORIENTED_EDGE ( 'NONE', *, *, #70209, .T. ) ;
#59559=EDGE_CURVE ( 'NONE', #91371, #57418, #45694, .T. ) ;
#59606=ORIENTED_EDGE ( 'NONE', *, *, #62730, .T. ) ;
#59620=CARTESIAN_POINT ( 'NONE',  ( -55.56624327025929944, 44.99999999999998579, 10.00000000000000000 ) ) ;
#59688=CARTESIAN_POINT ( 'NONE',  ( -110.0000000000000000, 0.000000000000000000, 59.99999999999999289 ) ) ;
#59735=VERTEX_POINT ( 'NONE', #46710 ) ;
#59753=ADVANCED_FACE ( 'NONE', ( #95238 ), #618, .F. ) ;
#59791=LINE ( 'NONE', #76509, #31866 ) ;
#59812=LINE ( 'NONE', #60792, #90396 ) ;
#59838=CARTESIAN_POINT ( 'NONE',  ( -13.11024591527734451, 0.000000000000000000, 45.00000000000000000 ) ) ;
#59862=CARTESIAN_POINT ( 'NONE',  ( -13.11024591527734451, 27.99999999999999645, 48.00000000000000000 ) ) ;
#59902=PLANE ( 'NONE',  #75845 ) ;
#59978=VECTOR ( 'NONE', #53323, 1000.000000000000000 ) ;
#59980=ORIENTED_EDGE ( 'NONE', *, *, #18521, .T. ) ;
#60003=ORIENTED_EDGE ( 'NONE', *, *, #34434, .F. ) ;
#60038=DIRECTION ( 'NONE',  ( -0.000000000000000000, 1.000000000000000000, -0.000000000000000000 ) ) ;
#60081=CARTESIAN_POINT ( 'NONE',  ( -19.65312891409030271, 9.999999999999994671, 54.99999999999999289 ) ) ;
#60117=AXIS2_PLACEMENT_3D ( 'NONE', #21502, #28589, #91426 ) ;
#60118=ORIENTED_EDGE ( 'NONE', *, *, #46263, .F. ) ;
#60148=VERTEX_POINT ( 'NONE', #45172 ) ;
#60212=DIRECTION ( 'NONE',  ( -0.000000000000000000, 0.000000000000000000, -1.000000000000000000 ) ) ;
#60227=EDGE_CURVE ( 'NONE', #30330, #9173, #49649, .T. ) ;
#60244=ORIENTED_EDGE ( 'NONE', *, *, #9599, .T. ) ;
#60345=PLANE ( 'NONE',  #40855 ) ;
#60367=ORIENTED_EDGE ( 'NONE', *, *, #43885, .T. ) ;
#60507=ORIENTED_EDGE ( 'NONE', *, *, #10312, .T. ) ;
#60530=VECTOR ( 'NONE', #47916, 1000.000000000000114 ) ;
#60534=LINE ( 'NONE', #86281, #73764 ) ;
#60585=CARTESIAN_POINT ( 'NONE',  ( 93.96857342517718337, 4.999999999999999112, 14.21260523776213347 ) ) ;
#60657=DIRECTION ( 'NONE',  ( -0.000000000000000000, 0.000000000000000000, -1.000000000000000000 ) ) ;
#60685=CARTESIAN_POINT ( 'NONE',  ( -19.65312891409030271, 93.06504152958497400, -59.99999999999999289 ) ) ;
#60724=ORIENTED_EDGE ( 'NONE', *, *, #79915, .T. ) ;
#60727=DIRECTION ( 'NONE',  ( 0.000000000000000000, 0.000000000000000000, 1.000000000000000000 ) ) ;
#60733=PRODUCT_DEFINITION_FORMATION_WITH_SPECIFIED_SOURCE ( 'ANY', '', #74307, .NOT_KNOWN. ) ;
#60771=AXIS2_PLACEMENT_3D ( 'NONE', #10992, #97115, #64680 ) ;
#60792=CARTESIAN_POINT ( 'NONE',  ( 49.80235952159635815, 85.00000000000000000, -10.00000000000000000 ) ) ;
#60826=CARTESIAN_POINT ( 'NONE',  ( 49.80235952159635104, 79.38263285747564169, 10.00000000000000000 ) ) ;
#60854=LINE ( 'NONE', #21391, #19329 ) ;
#60965=( LENGTH_UNIT ( ) NAMED_UNIT ( * ) SI_UNIT ( .MILLI., .METRE. ) );
#61006=EDGE_CURVE ( 'NONE', #91430, #79527, #46420, .T. ) ;
#61077=DIRECTION ( 'NONE',  ( -0.5000000000000016653, 0.8660254037844377084, 0.000000000000000000 ) ) ;
#61087=VECTOR ( 'NONE', #77611, 1000.000000000000000 ) ;
#61114=ORIENTED_EDGE ( 'NONE', *, *, #9599, .F. ) ;
#61117=VERTEX_POINT ( 'NONE', #23617 ) ;
#61123=DIRECTION ( 'NONE',  ( 0.000000000000000000, 0.000000000000000000, 1.000000000000000000 ) ) ;
#61184=DIRECTION ( 'NONE',  ( -0.000000000000000000, -0.000000000000000000, -1.000000000000000000 ) ) ;
#61222=VERTEX_POINT ( 'NONE', #58253 ) ;
#61226=ORIENTED_EDGE ( 'NONE', *, *, #86339, .T. ) ;
#61252=PLANE ( 'NONE',  #47828 ) ;
#61254=VECTOR ( 'NONE', #48755, 1000.000000000000000 ) ;
#61312=CARTESIAN_POINT ( 'NONE',  ( -57.77801984846012573, 31.16909059156539996, 59.99999999999999289 ) ) ;
#61359=ORIENTED_EDGE ( 'NONE', *, *, #74536, .F. ) ;
#61374=DIRECTION ( 'NONE',  ( -0.000000000000000000, -0.000000000000000000, -1.000000000000000000 ) ) ;
#61410=VERTEX_POINT ( 'NONE', #13180 ) ;
#61427=CARTESIAN_POINT ( 'NONE',  ( -105.0000000000000000, 10.00000000000000000, -14.21260523776212281 ) ) ;
#61429=DIRECTION ( 'NONE',  ( 0.000000000000000000, 0.000000000000000000, 1.000000000000000000 ) ) ;
#61436=VERTEX_POINT ( 'NONE', #89713 ) ;
#61648=ORIENTED_EDGE ( 'NONE', *, *, #99241, .F. ) ;
#61667=LINE ( 'NONE', #7991, #17337 ) ;
#61740=EDGE_CURVE ( 'NONE', #98779, #21265, #36834, .T. ) ;
#61753=CARTESIAN_POINT ( 'NONE',  ( 79.99999999999997158, 26.16025403784438907, 59.99999999999999289 ) ) ;
#61780=VERTEX_POINT ( 'NONE', #59620 ) ;
#61807=ORIENTED_EDGE ( 'NONE', *, *, #37610, .T. ) ;
#61810=PLANE ( 'NONE',  #90647 ) ;
#61823=ADVANCED_FACE ( 'NONE', ( #68224 ), #4960, .T. ) ;
#61960=CARTESIAN_POINT ( 'NONE',  ( 79.99999999999998579, 20.00000000000000000, 59.99999999999999289 ) ) ;
#62266=LINE ( 'NONE', #55170, #88228 ) ;
#62286=DIRECTION ( 'NONE',  ( 0.000000000000000000, -1.000000000000000000, 0.000000000000000000 ) ) ;
#62328=CARTESIAN_POINT ( 'NONE',  ( -105.0000000000000000, 9.999999999999998224, 59.99999999999999289 ) ) ;
#62337=ORIENTED_EDGE ( 'NONE', *, *, #50360, .F. ) ;
#62342=PLANE ( 'NONE',  #19845 ) ;
#62411=ORIENTED_EDGE ( 'NONE', *, *, #93233, .F. ) ;
#62449=( NAMED_UNIT ( * ) SI_UNIT ( $, .STERADIAN. ) SOLID_ANGLE_UNIT ( ) );
#62537=VECTOR ( 'NONE', #30931, 1000.000000000000000 ) ;
#62570=AXIS2_PLACEMENT_3D ( 'NONE', #43192, #4729, #97437 ) ;
#62578=VECTOR ( 'NONE', #7952, 1000.000000000000000 ) ;
#62634=CARTESIAN_POINT ( 'NONE',  ( -13.11024591527734451, 0.000000000000000000, -20.00000000000000000 ) ) ;
#62658=FACE_BOUND ( 'NONE', #37647, .T. ) ;
#62730=EDGE_CURVE ( 'NONE', #31854, #91585, #49027, .T. ) ;
#62732=CARTESIAN_POINT ( 'NONE',  ( -13.11024591527734451, 6.000000000000000000, 40.00000000000000000 ) ) ;
#62833=CARTESIAN_POINT ( 'NONE',  ( -86.81108781737714253, -8.000000000000000000, -14.21260523776213347 ) ) ;
#62916=ORIENTED_EDGE ( 'NONE', *, *, #77834, .F. ) ;
#62961=DIRECTION ( 'NONE',  ( 0.000000000000000000, -1.000000000000000000, 0.000000000000000000 ) ) ;
#63022=CARTESIAN_POINT ( 'NONE',  ( 51.80235952159637236, 80.00000000000000000, 59.99999999999999289 ) ) ;
#63029=PLANE ( 'NONE',  #65997 ) ;
#63095=LINE ( 'NONE', #54472, #42583 ) ;
#63115=DIRECTION ( 'NONE',  ( -0.000000000000000000, 1.000000000000000000, -0.000000000000000000 ) ) ;
#63123=CYLINDRICAL_SURFACE ( 'NONE', #89939, 7.499999999999992895 ) ;
#63129=ORIENTED_EDGE ( 'NONE', *, *, #81797, .F. ) ;
#63247=CARTESIAN_POINT ( 'NONE',  ( -110.0000000000000000, 0.000000000000000000, 59.99999999999999289 ) ) ;
#63265=CARTESIAN_POINT ( 'NONE',  ( -21.44506416300749407, 94.09961582791768819, -54.99999999999999289 ) ) ;
#63281=ORIENTED_EDGE ( 'NONE', *, *, #76180, .F. ) ;
#63349=ORIENTED_EDGE ( 'NONE', *, *, #23207, .F. ) ;
#63371=ORIENTED_EDGE ( 'NONE', *, *, #50742, .T. ) ;
#63378=CARTESIAN_POINT ( 'NONE',  ( -13.11024591527723615, 27.99999999999999645, -32.50000000000017053 ) ) ;
#63442=FACE_OUTER_BOUND ( 'NONE', #1695, .T. ) ;
#63496=FACE_OUTER_BOUND ( 'NONE', #40808, .T. ) ;
#63519=DIRECTION ( 'NONE',  ( 0.000000000000000000, -1.000000000000000000, 0.000000000000000000 ) ) ;
#63528=FACE_OUTER_BOUND ( 'NONE', #8205, .T. ) ;
#63587=LINE ( 'NONE', #94528, #39240 ) ;
#63624=VERTEX_POINT ( 'NONE', #11554 ) ;
#63728=DIRECTION ( 'NONE',  ( -0.000000000000000000, -1.000000000000000000, -0.000000000000000000 ) ) ;
#63778=ORIENTED_EDGE ( 'NONE', *, *, #83384, .F. ) ;
#63796=DIRECTION ( 'NONE',  ( -0.000000000000000000, 1.000000000000000000, -0.000000000000000000 ) ) ;
#63863=FACE_OUTER_BOUND ( 'NONE', #10074, .T. ) ;
#63868=ORIENTED_EDGE ( 'NONE', *, *, #71457, .T. ) ;
#63901=LINE ( 'NONE', #3142, #17039 ) ;
#63981=DIRECTION ( 'NONE',  ( 0.000000000000000000, 0.000000000000000000, -1.000000000000000000 ) ) ;
#63991=VERTEX_POINT ( 'NONE', #809 ) ;
#64006=EDGE_LOOP ( 'NONE', ( #2349, #50840 ) ) ;
#64077=CARTESIAN_POINT ( 'NONE',  ( -19.65312891409030271, 93.06504152958497400, 10.00000000000000000 ) ) ;
#64126=EDGE_CURVE ( 'NONE', #49525, #3243, #12934, .T. ) ;
#64150=AXIS2_PLACEMENT_3D ( 'NONE', #13090, #82528, #33902 ) ;
#64222=AXIS2_PLACEMENT_3D ( 'NONE', #27636, #36200, #58501 ) ;
#64266=LINE ( 'NONE', #93708, #35032 ) ;
#64308=ORIENTED_EDGE ( 'NONE', *, *, #51867, .F. ) ;
#64328=VECTOR ( 'NONE', #42605, 1000.000000000000000 ) ;
#64385=VERTEX_POINT ( 'NONE', #27144 ) ;
#64469=VECTOR ( 'NONE', #76037, 1000.000000000000000 ) ;
#64503=ORIENTED_EDGE ( 'NONE', *, *, #44455, .T. ) ;
#64605=LINE ( 'NONE', #35186, #99247 ) ;
#64628=AXIS2_PLACEMENT_3D ( 'NONE', #31177, #93529, #61077 ) ;
#64680=DIRECTION ( 'NONE',  ( 0.000000000000000000, 0.000000000000000000, 1.000000000000000000 ) ) ;
#64698=AXIS2_PLACEMENT_3D ( 'NONE', #39809, #56015, #93066 ) ;
#64710=ADVANCED_FACE ( 'NONE', ( #96455 ), #2737, .F. ) ;
#64731=CYLINDRICAL_SURFACE ( 'NONE', #40980, 12.49999999999999645 ) ;
#64759=FACE_OUTER_BOUND ( 'NONE', #13545, .T. ) ;
#64760=LINE ( 'NONE', #96189, #72481 ) ;
#64869=DIRECTION ( 'NONE',  ( -0.000000000000000000, -1.000000000000000000, -0.000000000000000000 ) ) ;
#64973=LINE ( 'NONE', #42151, #87102 ) ;
#64991=CARTESIAN_POINT ( 'NONE',  ( 84.99999999999998579, 14.99999999999999467, 59.99999999999999289 ) ) ;
#65021=DIRECTION ( 'NONE',  ( 1.000000000000000000, 0.000000000000000000, 0.000000000000000000 ) ) ;
#65026=EDGE_CURVE ( 'NONE', #58073, #49297, #87768, .T. ) ;
#65086=LINE ( 'NONE', #3799, #1530 ) ;
#65117=VERTEX_POINT ( 'NONE', #67376 ) ;
#65259=FACE_OUTER_BOUND ( 'NONE', #42017, .T. ) ;
#65398=FACE_OUTER_BOUND ( 'NONE', #44458, .T. ) ;
#65491=CARTESIAN_POINT ( 'NONE',  ( -105.0000000000000000, 0.000000000000000000, 59.99999999999999289 ) ) ;
#65519=CARTESIAN_POINT ( 'NONE',  ( 13.52134341065866430, 31.30466486950697558, 0.000000000000000000 ) ) ;
#65530=VECTOR ( 'NONE', #20806, 1000.000000000000000 ) ;
#65586=ORIENTED_EDGE ( 'NONE', *, *, #35325, .F. ) ;
#65750=VERTEX_POINT ( 'NONE', #96852 ) ;
#65765=ORIENTED_EDGE ( 'NONE', *, *, #78809, .T. ) ;
#65857=EDGE_LOOP ( 'NONE', ( #75512, #46727, #3148, #27092 ) ) ;
#65977=DIRECTION ( 'NONE',  ( -1.000000000000000000, -1.110223024625156343E-15, 0.000000000000000000 ) ) ;
#65997=AXIS2_PLACEMENT_3D ( 'NONE', #39204, #55405, #47811 ) ;
#66011=ORIENTED_EDGE ( 'NONE', *, *, #40283, .F. ) ;
#66078=EDGE_CURVE ( 'NONE', #14428, #13682, #15497, .T. ) ;
#66150=CIRCLE ( 'NONE', #83977, 9.212605237762131694 ) ;
#66152=ORIENTED_EDGE ( 'NONE', *, *, #53077, .T. ) ;
#66195=LINE ( 'NONE', #96639, #16792 ) ;
#66230=CYLINDRICAL_SURFACE ( 'NONE', #27852, 12.50000000000000000 ) ;
#66278=ORIENTED_EDGE ( 'NONE', *, *, #98872, .T. ) ;
#66309=LINE ( 'NONE', #29800, #41495 ) ;
#66318=ORIENTED_EDGE ( 'NONE', *, *, #52325, .F. ) ;
#66356=DIRECTION ( 'NONE',  ( -0.4999999999999997780, -0.8660254037844387076, 0.000000000000000000 ) ) ;
#66415=ORIENTED_EDGE ( 'NONE', *, *, #50360, .T. ) ;
#66426=ADVANCED_FACE ( 'NONE', ( #21032, #99517 ), #51404, .T. ) ;
#66472=ORIENTED_EDGE ( 'NONE', *, *, #24734, .F. ) ;
#66475=ORIENTED_EDGE ( 'NONE', *, *, #355, .F. ) ;
#66506=CARTESIAN_POINT ( 'NONE',  ( -13.11024591527734628, 27.99999999999999645, 32.50000000000000000 ) ) ;
#66511=DIRECTION ( 'NONE',  ( 0.000000000000000000, 1.000000000000000000, 0.000000000000000000 ) ) ;
#66544=CARTESIAN_POINT ( 'NONE',  ( 93.96857342517718337, 15.00000000000000000, -9.212605237762131694 ) ) ;
#66674=EDGE_CURVE ( 'NONE', #59735, #87466, #66150, .T. ) ;
#66689=DIRECTION ( 'NONE',  ( 0.000000000000000000, -1.000000000000000000, 0.000000000000000000 ) ) ;
#66765=ADVANCED_FACE ( 'NONE', ( #54245 ), #85218, .F. ) ;
#66815=CARTESIAN_POINT ( 'NONE',  ( 39.80235952159635815, 84.99999999999998579, 10.00000000000000000 ) ) ;
#66880=ORIENTED_EDGE ( 'NONE', *, *, #26764, .T. ) ;
#66906=DIRECTION ( 'NONE',  ( 0.000000000000000000, 0.000000000000000000, 1.000000000000000000 ) ) ;
#66911=CARTESIAN_POINT ( 'NONE',  ( -13.11024591527723615, 27.99999999999999645, -48.00000000000017053 ) ) ;
#66918=DIRECTION ( 'NONE',  ( 1.235257323912246174E-15, 1.000000000000000000, -0.000000000000000000 ) ) ;
#67017=CARTESIAN_POINT ( 'NONE',  ( 84.99999999999998579, 14.99999999999999467, 59.99999999999999289 ) ) ;
#67032=APPLICATION_CONTEXT ( 'automotive_design' ) ;
#67037=CARTESIAN_POINT ( 'NONE',  ( -13.11024591527734628, 4.999999999999999112, 17.00000000000000000 ) ) ;
#67081=ORIENTED_EDGE ( 'NONE', *, *, #51867, .T. ) ;
#67160=DIRECTION ( 'NONE',  ( -0.000000000000000000, -1.000000000000000000, -0.000000000000000000 ) ) ;
#67292=VECTOR ( 'NONE', #20974, 1000.000000000000000 ) ;
#67367=EDGE_LOOP ( 'NONE', ( #94599, #72036, #67081, #55162 ) ) ;
#67376=CARTESIAN_POINT ( 'NONE',  ( 93.96857342517718337, 0.000000000000000000, -9.212605237762131694 ) ) ;
#67426=AXIS2_PLACEMENT_3D ( 'NONE', #93119, #56064, #891 ) ;
#67490=ORIENTED_EDGE ( 'NONE', *, *, #78427, .F. ) ;
#67512=LINE ( 'NONE', #74653, #1015 ) ;
#67598=CARTESIAN_POINT ( 'NONE',  ( -65.00000000000000000, 93.06504152958497400, -54.99999999999999289 ) ) ;
#67613=ORIENTED_EDGE ( 'NONE', *, *, #55531, .F. ) ;
#67617=EDGE_LOOP ( 'NONE', ( #58513, #91053 ) ) ;
#67627=ORIENTED_EDGE ( 'NONE', *, *, #28077, .F. ) ;
#67789=DIRECTION ( 'NONE',  ( -1.000000000000000000, 0.000000000000000000, 0.000000000000000000 ) ) ;
#67829=EDGE_CURVE ( 'NONE', #17199, #41822, #18965, .T. ) ;
#67889=LINE ( 'NONE', #28379, #65530 ) ;
#67933=AXIS2_PLACEMENT_3D ( 'NONE', #93964, #63519, #76725 ) ;
#67970=FACE_OUTER_BOUND ( 'NONE', #33364, .T. ) ;
#67993=ORIENTED_EDGE ( 'NONE', *, *, #16047, .F. ) ;
#67999=ORIENTED_EDGE ( 'NONE', *, *, #7207, .F. ) ;
#68080=DIRECTION ( 'NONE',  ( 0.000000000000000000, -0.000000000000000000, 1.000000000000000000 ) ) ;
#68088=FACE_BOUND ( 'NONE', #58609, .T. ) ;
#68139=EDGE_LOOP ( 'NONE', ( #26782, #3110, #61114, #71248, #97802, #27257, #34691, #70730, #56503, #90875, #4184 ) ) ;
#68224=FACE_OUTER_BOUND ( 'NONE', #78346, .T. ) ;
#68342=EDGE_LOOP ( 'NONE', ( #33913, #82102, #32326, #29018, #76486, #93318, #48673, #57615, #95959, #1783, #25754 ) ) ;
#68356=FACE_OUTER_BOUND ( 'NONE', #28462, .T. ) ;
#68439=DIRECTION ( 'NONE',  ( 0.000000000000000000, 0.000000000000000000, 1.000000000000000000 ) ) ;
#68546=VECTOR ( 'NONE', #93281, 1000.000000000000000 ) ;
#68626=CARTESIAN_POINT ( 'NONE',  ( -65.66987298107781612, 17.49999999999999645, 10.00000000000000178 ) ) ;
#68698=( GEOMETRIC_REPRESENTATION_CONTEXT ( 3 ) GLOBAL_UNCERTAINTY_ASSIGNED_CONTEXT ( ( #33154 ) ) GLOBAL_UNIT_ASSIGNED_CONTEXT ( ( #20316, #25927, #22291 ) ) REPRESENTATION_CONTEXT ( 'NONE', 'WORKASPACE' ) );
#68741=ORIENTED_EDGE ( 'NONE', *, *, #15010, .F. ) ;
#68778=LINE ( 'NONE', #76879, #70555 ) ;
#68784=AXIS2_PLACEMENT_3D ( 'NONE', #15354, #91924, #23457 ) ;
#68895=EDGE_CURVE ( 'NONE', #61117, #100286, #55201, .T. ) ;
#68898=PLANE ( 'NONE',  #12578 ) ;
#68927=EDGE_CURVE ( 'NONE', #75741, #69092, #84660, .T. ) ;
#68936=CARTESIAN_POINT ( 'NONE',  ( 49.80235952159635104, 79.38263285747564169, -10.00000000000000000 ) ) ;
#68944=VECTOR ( 'NONE', #69258, 1000.000000000000000 ) ;
#68955=CARTESIAN_POINT ( 'NONE',  ( 35.39012114306879653, 16.59285393851897084, -10.00000000000000000 ) ) ;
#68975=VECTOR ( 'NONE', #33500, 1000.000000000000000 ) ;
#69092=VERTEX_POINT ( 'NONE', #27816 ) ;
#69124=EDGE_LOOP ( 'NONE', ( #85336, #3867, #24746, #35593 ) ) ;
#69164=CARTESIAN_POINT ( 'NONE',  ( -86.81108781737714253, 10.00000000000000178, 14.21260523776213347 ) ) ;
#69212=ORIENTED_EDGE ( 'NONE', *, *, #21787, .T. ) ;
#69243=AXIS2_PLACEMENT_3D ( 'NONE', #96998, #81786, #34645 ) ;
#69258=DIRECTION ( 'NONE',  ( -1.000000000000000000, -1.156482317317871331E-15, 0.000000000000000000 ) ) ;
#69348=DIRECTION ( 'NONE',  ( -0.000000000000000000, -1.000000000000000000, -0.000000000000000000 ) ) ;
#69368=ORIENTED_EDGE ( 'NONE', *, *, #58367, .F. ) ;
#69455=VECTOR ( 'NONE', #25457, 1000.000000000000000 ) ;
#69475=EDGE_CURVE ( 'NONE', #2827, #17355, #44997, .T. ) ;
#69508=EDGE_CURVE ( 'NONE', #89960, #7425, #41646, .T. ) ;
#69529=CARTESIAN_POINT ( 'NONE',  ( -13.11024591527723615, 6.000000000000000000, -40.00000000000016342 ) ) ;
#69704=ORIENTED_EDGE ( 'NONE', *, *, #37494, .F. ) ;
#69773=CARTESIAN_POINT ( 'NONE',  ( -13.11024591527723615, 27.99999999999999645, -32.50000000000017053 ) ) ;
#69782=CARTESIAN_POINT ( 'NONE',  ( 93.96857342517719758, 4.999999999999999112, 0.000000000000000000 ) ) ;
#69821=ORIENTED_EDGE ( 'NONE', *, *, #55656, .F. ) ;
#69856=ORIENTED_EDGE ( 'NONE', *, *, #71939, .F. ) ;
#69898=DIRECTION ( 'NONE',  ( -5.984665299743594308E-16, 0.000000000000000000, -1.000000000000000000 ) ) ;
#69915=DIRECTION ( 'NONE',  ( 0.5000000000000011102, 0.8660254037844380415, 0.000000000000000000 ) ) ;
#69960=VERTEX_POINT ( 'NONE', #55325 ) ;
#70082=DIRECTION ( 'NONE',  ( 0.000000000000000000, 1.000000000000000000, 0.000000000000000000 ) ) ;
#70143=FACE_OUTER_BOUND ( 'NONE', #51287, .T. ) ;
#70179=DIRECTION ( 'NONE',  ( -1.000000000000000000, 0.000000000000000000, 0.000000000000000000 ) ) ;
#70209=EDGE_CURVE ( 'NONE', #76847, #98779, #91286, .T. ) ;
#70320=EDGE_LOOP ( 'NONE', ( #34367, #43677, #63129, #15179 ) ) ;
#70362=ORIENTED_EDGE ( 'NONE', *, *, #12211, .F. ) ;
#70397=FACE_OUTER_BOUND ( 'NONE', #31830, .T. ) ;
#70421=EDGE_LOOP ( 'NONE', ( #52782, #38194, #58159, #86607, #19056 ) ) ;
#70470=PLANE ( 'NONE',  #79141 ) ;
#70486=CARTESIAN_POINT ( 'NONE',  ( -19.65312891409030271, 93.06504152958497400, -10.00000000000000000 ) ) ;
#70555=VECTOR ( 'NONE', #38370, 1000.000000000000000 ) ;
#70609=EDGE_LOOP ( 'NONE', ( #11193, #36865, #88760, #78085 ) ) ;
#70730=ORIENTED_EDGE ( 'NONE', *, *, #6026, .F. ) ;
#70744=EDGE_LOOP ( 'NONE', ( #95460, #43743 ) ) ;
#70757=ADVANCED_FACE ( 'NONE', ( #28847 ), #51648, .F. ) ;
#70838=ORIENTED_EDGE ( 'NONE', *, *, #55531, .T. ) ;
#70957=CIRCLE ( 'NONE', #83932, 12.50000000000000000 ) ;
#70982=ORIENTED_EDGE ( 'NONE', *, *, #59092, .T. ) ;
#70991=ORIENTED_EDGE ( 'NONE', *, *, #20153, .T. ) ;
#71080=ORIENTED_EDGE ( 'NONE', *, *, #16047, .T. ) ;
#71143=CIRCLE ( 'NONE', #27455, 7.499999999999996447 ) ;
#71217=CARTESIAN_POINT ( 'NONE',  ( 93.96857342517719758, 0.000000000000000000, 0.000000000000000000 ) ) ;
#71226=VECTOR ( 'NONE', #57436, 1000.000000000000000 ) ;
#71248=ORIENTED_EDGE ( 'NONE', *, *, #62730, .F. ) ;
#71293=PRODUCT_DEFINITION ( 'UNKNOWN', '', #60733, #17975 ) ;
#71309=FACE_BOUND ( 'NONE', #8199, .T. ) ;
#71332=DIRECTION ( 'NONE',  ( 1.000000000000000000, 0.000000000000000000, 0.000000000000000000 ) ) ;
#71384=EDGE_LOOP ( 'NONE', ( #43623, #54247, #24789, #18906 ) ) ;
#71414=DIRECTION ( 'NONE',  ( -1.804112415015878984E-15, 1.000000000000000000, -0.000000000000000000 ) ) ;
#71457=EDGE_CURVE ( 'NONE', #38156, #6816, #3421, .T. ) ;
#71482=EDGE_CURVE ( 'NONE', #89960, #38156, #1906, .T. ) ;
#71540=DIRECTION ( 'NONE',  ( -1.000000000000000000, 0.000000000000000000, 0.000000000000000000 ) ) ;
#71551=VECTOR ( 'NONE', #100265, 1000.000000000000000 ) ;
#71580=CARTESIAN_POINT ( 'NONE',  ( -13.11024591527734628, 0.000000000000000000, 32.50000000000000000 ) ) ;
#71611=CARTESIAN_POINT ( 'NONE',  ( -65.00000000000000000, 18.66025403784439973, 59.99999999999999289 ) ) ;
#71623=DIRECTION ( 'NONE',  ( -1.000000000000000000, 0.000000000000000000, 0.000000000000000000 ) ) ;
#71645=LINE ( 'NONE', #89375, #57434 ) ;
#71668=ORIENTED_EDGE ( 'NONE', *, *, #66674, .F. ) ;
#71688=CYLINDRICAL_SURFACE ( 'NONE', #88832, 7.500000000000000000 ) ;
#71757=ORIENTED_EDGE ( 'NONE', *, *, #29469, .T. ) ;
#71888=ADVANCED_FACE ( 'NONE', ( #86436 ), #8871, .F. ) ;
#71912=LINE ( 'NONE', #24302, #1061 ) ;
#71939=EDGE_CURVE ( 'NONE', #61410, #79692, #28967, .T. ) ;
#71983=ORIENTED_EDGE ( 'NONE', *, *, #68927, .T. ) ;
#72036=ORIENTED_EDGE ( 'NONE', *, *, #18521, .F. ) ;
#72201=LINE ( 'NONE', #96026, #8699 ) ;
#72254=VECTOR ( 'NONE', #16057, 1000.000000000000000 ) ;
#72267=DIRECTION ( 'NONE',  ( 0.000000000000000000, 0.000000000000000000, 1.000000000000000000 ) ) ;
#72466=LINE ( 'NONE', #3071, #13701 ) ;
#72481=VECTOR ( 'NONE', #17142, 1000.000000000000000 ) ;
#72575=CIRCLE ( 'NONE', #75825, 15.50000000000000000 ) ;
#72612=AXIS2_PLACEMENT_3D ( 'NONE', #29119, #6802, #13904 ) ;
#72696=CIRCLE ( 'NONE', #96937, 9.212605237762131694 ) ;
#72740=ADVANCED_FACE ( 'NONE', ( #83435 ), #46366, .F. ) ;
#72845=LINE ( 'NONE', #33313, #9471 ) ;
#73097=DIRECTION ( 'NONE',  ( -0.5000000000000014433, 0.8660254037844379305, 0.000000000000000000 ) ) ;
#73122=ORIENTED_EDGE ( 'NONE', *, *, #22287, .T. ) ;
#73127=ORIENTED_EDGE ( 'NONE', *, *, #59099, .T. ) ;
#73165=CARTESIAN_POINT ( 'NONE',  ( 39.80235952159635815, 84.99999999999998579, -10.00000000000000000 ) ) ;
#73204=ADVANCED_FACE ( 'NONE', ( #87845 ), #32057, .F. ) ;
#73236=DIRECTION ( 'NONE',  ( -0.000000000000000000, 1.000000000000000000, -0.000000000000000000 ) ) ;
#73250=CARTESIAN_POINT ( 'NONE',  ( 110.0000000000000000, -8.000000000000000000, -14.21260523776213347 ) ) ;
#73320=EDGE_CURVE ( 'NONE', #53652, #58927, #71143, .T. ) ;
#73356=VECTOR ( 'NONE', #97640, 1000.000000000000000 ) ;
#73410=CARTESIAN_POINT ( 'NONE',  ( -13.11024591527723437, 27.99999999999999645, -17.00000000000016698 ) ) ;
#73434=ADVANCED_FACE ( 'NONE', ( #68356 ), #97422, .F. ) ;
#73508=EDGE_LOOP ( 'NONE', ( #77892, #81251, #99882, #90363, #200, #2134, #80271, #63778 ) ) ;
#73592=PLANE ( 'NONE',  #2552 ) ;
#73637=ORIENTED_EDGE ( 'NONE', *, *, #89062, .T. ) ;
#73665=ORIENTED_EDGE ( 'NONE', *, *, #29165, .T. ) ;
#73715=CARTESIAN_POINT ( 'NONE',  ( -13.11024591527734628, 6.000000000000000000, -32.50000000000000000 ) ) ;
#73721=ADVANCED_FACE ( 'NONE', ( #17032 ), #47433, .F. ) ;
#73764=VECTOR ( 'NONE', #60038, 1000.000000000000000 ) ;
#73777=FACE_OUTER_BOUND ( 'NONE', #59204, .T. ) ;
#73820=LINE ( 'NONE', #35308, #73356 ) ;
#73847=CARTESIAN_POINT ( 'NONE',  ( 79.99999999999997158, 26.16025403784438907, -54.99999999999999289 ) ) ;
#73888=EDGE_CURVE ( 'NONE', #26545, #5700, #11352, .T. ) ;
#73963=VECTOR ( 'NONE', #15305, 1000.000000000000114 ) ;
#74040=AXIS2_PLACEMENT_3D ( 'NONE', #30907, #69898, #512 ) ;
#74047=LINE ( 'NONE', #35529, #4646 ) ;
#74129=CYLINDRICAL_SURFACE ( 'NONE', #26649, 15.50000000000000000 ) ;
#74133=CARTESIAN_POINT ( 'NONE',  ( -65.00000000000000000, 10.00000000000000000, 54.99999999999999289 ) ) ;
#74136=FACE_BOUND ( 'NONE', #5699, .T. ) ;
#74160=CIRCLE ( 'NONE', #28868, 10.00000000000001066 ) ;
#74227=EDGE_CURVE ( 'NONE', #79527, #2619, #90627, .T. ) ;
#74236=EDGE_CURVE ( 'NONE', #97401, #88729, #79771, .T. ) ;
#74254=ORIENTED_EDGE ( 'NONE', *, *, #18587, .F. ) ;
#74270=DIRECTION ( 'NONE',  ( 0.000000000000000000, 1.000000000000000000, 0.000000000000000000 ) ) ;
#74305=CARTESIAN_POINT ( 'NONE',  ( -105.0000000000000000, 10.00000000000000000, -54.99999999999999289 ) ) ;
#74306=ORIENTED_EDGE ( 'NONE', *, *, #19017, .F. ) ;
#74307=PRODUCT ( 'Lower Tilting Cradle Base Segment', 'Lower Tilting Cradle Base Segment', '', ( #46129 ) ) ;
#74354=VECTOR ( 'NONE', #26267, 1000.000000000000000 ) ;
#74374=VECTOR ( 'NONE', #39024, 1000.000000000000000 ) ;
#74381=CARTESIAN_POINT ( 'NONE',  ( -51.42721978966704910, 42.16899896210639298, -54.99999999999999289 ) ) ;
#74536=EDGE_CURVE ( 'NONE', #94434, #98779, #39572, .T. ) ;
#74579=ADVANCED_FACE ( 'NONE', ( #65398 ), #57289, .T. ) ;
#74611=LINE ( 'NONE', #59862, #54641 ) ;
#74653=CARTESIAN_POINT ( 'NONE',  ( 35.39012114306879653, 16.59285393851897084, -10.00000000000000000 ) ) ;
#74677=FACE_OUTER_BOUND ( 'NONE', #44680, .T. ) ;
#74705=CARTESIAN_POINT ( 'NONE',  ( -13.11024591527734628, 15.00000000000000000, 25.00000000000000000 ) ) ;
#74759=FACE_OUTER_BOUND ( 'NONE', #93561, .T. ) ;
#74828=DIRECTION ( 'NONE',  ( -0.5000000000000014433, 0.8660254037844379305, 0.000000000000000000 ) ) ;
#74893=CARTESIAN_POINT ( 'NONE',  ( -21.44506416300749407, 94.09961582791768819, 54.99999999999999289 ) ) ;
#74902=ORIENTED_EDGE ( 'NONE', *, *, #43091, .T. ) ;
#74909=PLANE ( 'NONE',  #28973 ) ;
#75142=EDGE_CURVE ( 'NONE', #35859, #43346, #26493, .T. ) ;
#75171=AXIS2_PLACEMENT_3D ( 'NONE', #40651, #56355, #1688 ) ;
#75345=ORIENTED_EDGE ( 'NONE', *, *, #55656, .T. ) ;
#75360=DIRECTION ( 'NONE',  ( 1.082076799516502080E-16, 0.000000000000000000, 1.000000000000000000 ) ) ;
#75404=LINE ( 'NONE', #92138, #37054 ) ;
#75424=EDGE_CURVE ( 'NONE', #33343, #91371, #56656, .T. ) ;
#75447=ORIENTED_EDGE ( 'NONE', *, *, #29165, .F. ) ;
#75468=EDGE_CURVE ( 'NONE', #22518, #6816, #18100, .T. ) ;
#75512=ORIENTED_EDGE ( 'NONE', *, *, #795, .F. ) ;
#75516=DIRECTION ( 'NONE',  ( -1.000000000000000000, 0.000000000000000000, 0.000000000000000000 ) ) ;
#75521=VERTEX_POINT ( 'NONE', #92984 ) ;
#75528=FACE_OUTER_BOUND ( 'NONE', #70744, .T. ) ;
#75534=CARTESIAN_POINT ( 'NONE',  ( -86.81108781737714253, 10.00000000000000178, -14.21260523776213347 ) ) ;
#75564=FACE_OUTER_BOUND ( 'NONE', #71384, .T. ) ;
#75575=CARTESIAN_POINT ( 'NONE',  ( -51.42721978966704910, 42.16899896210639298, 54.99999999999999289 ) ) ;
#75582=ORIENTED_EDGE ( 'NONE', *, *, #69508, .T. ) ;
#75660=LINE ( 'NONE', #45237, #5873 ) ;
#75663=VECTOR ( 'NONE', #51473, 1000.000000000000000 ) ;
#75665=ORIENTED_EDGE ( 'NONE', *, *, #18904, .F. ) ;
#75741=VERTEX_POINT ( 'NONE', #28539 ) ;
#75745=VECTOR ( 'NONE', #10552, 1000.000000000000000 ) ;
#75746=LINE ( 'NONE', #91975, #44890 ) ;
#75767=ORIENTED_EDGE ( 'NONE', *, *, #83875, .T. ) ;
#75799=EDGE_CURVE ( 'NONE', #48468, #2734, #20976, .T. ) ;
#75825=AXIS2_PLACEMENT_3D ( 'NONE', #52090, #83036, #21698 ) ;
#75845=AXIS2_PLACEMENT_3D ( 'NONE', #21422, #6715, #98935 ) ;
#75898=CARTESIAN_POINT ( 'NONE',  ( -105.0000000000000000, 4.999999999999999112, -14.21260523776212281 ) ) ;
#75919=AXIS2_PLACEMENT_3D ( 'NONE', #85390, #83894, #30142 ) ;
#75970=CARTESIAN_POINT ( 'NONE',  ( -19.65312891409030271, 93.06504152958497400, 59.99999999999999289 ) ) ;
#75980=ORIENTED_EDGE ( 'NONE', *, *, #75799, .F. ) ;
#76018=VERTEX_POINT ( 'NONE', #61427 ) ;
#76031=DIRECTION ( 'NONE',  ( -0.000000000000000000, -0.000000000000000000, -1.000000000000000000 ) ) ;
#76037=DIRECTION ( 'NONE',  ( -0.000000000000000000, 1.000000000000000000, -0.000000000000000000 ) ) ;
#76038=CARTESIAN_POINT ( 'NONE',  ( -110.0000000000000000, 0.000000000000000000, 59.99999999999999289 ) ) ;
#76117=EDGE_LOOP ( 'NONE', ( #36435, #97406 ) ) ;
#76125=DIRECTION ( 'NONE',  ( 1.235257323912246174E-15, 1.000000000000000000, 0.000000000000000000 ) ) ;
#76180=EDGE_CURVE ( 'NONE', #34316, #35306, #13122, .T. ) ;
#76245=ORIENTED_EDGE ( 'NONE', *, *, #58080, .T. ) ;
#76323=ORIENTED_EDGE ( 'NONE', *, *, #77682, .T. ) ;
#76363=CARTESIAN_POINT ( 'NONE',  ( -19.65312891409030271, 93.06504152958497400, 54.99999999999999289 ) ) ;
#76405=DIRECTION ( 'NONE',  ( 0.8575671445351807920, -0.5143720371616018472, 0.000000000000000000 ) ) ;
#76463=VECTOR ( 'NONE', #83581, 1000.000000000000000 ) ;
#76486=ORIENTED_EDGE ( 'NONE', *, *, #75142, .T. ) ;
#76509=CARTESIAN_POINT ( 'NONE',  ( -110.0000000000000000, 4.999999999999999112, 14.21260523776215301 ) ) ;
#76517=CARTESIAN_POINT ( 'NONE',  ( 93.96857342517718337, -8.000000000000000000, -14.21260523776213347 ) ) ;
#76522=ORIENTED_EDGE ( 'NONE', *, *, #36288, .T. ) ;
#76583=DIRECTION ( 'NONE',  ( 1.000000000000000000, 0.000000000000000000, 0.000000000000000000 ) ) ;
#76591=VERTEX_POINT ( 'NONE', #83337 ) ;
#76675=CARTESIAN_POINT ( 'NONE',  ( 93.96857342517718337, 10.00000000000001243, 14.21260523776213347 ) ) ;
#76696=ORIENTED_EDGE ( 'NONE', *, *, #20552, .T. ) ;
#76724=EDGE_CURVE ( 'NONE', #69960, #76591, #92921, .T. ) ;
#76725=DIRECTION ( 'NONE',  ( 0.000000000000000000, 0.000000000000000000, 1.000000000000000000 ) ) ;
#76741=ORIENTED_EDGE ( 'NONE', *, *, #39187, .F. ) ;
#76753=LINE ( 'NONE', #7346, #949 ) ;
#76825=LINE ( 'NONE', #47786, #82189 ) ;
#76845=ORIENTED_EDGE ( 'NONE', *, *, #7524, .F. ) ;
#76847=VERTEX_POINT ( 'NONE', #39662 ) ;
#76879=CARTESIAN_POINT ( 'NONE',  ( -57.04299263576977097, 30.72821847190685673, 10.00000000000000000 ) ) ;
#76976=DIRECTION ( 'NONE',  ( 1.000000000000000000, 1.156482317317871331E-15, 0.000000000000000000 ) ) ;
#77014=DIRECTION ( 'NONE',  ( -0.5000000000000014433, 0.8660254037844379305, 0.000000000000000000 ) ) ;
#77081=VERTEX_POINT ( 'NONE', #98226 ) ;
#77106=EDGE_LOOP ( 'NONE', ( #13402, #44307, #33232, #61226 ) ) ;
#77134=VECTOR ( 'NONE', #27034, 1000.000000000000000 ) ;
#77171=FACE_OUTER_BOUND ( 'NONE', #33848, .T. ) ;
#77204=ORIENTED_EDGE ( 'NONE', *, *, #46654, .T. ) ;
#77255=ORIENTED_EDGE ( 'NONE', *, *, #8799, .F. ) ;
#77334=ORIENTED_EDGE ( 'NONE', *, *, #54639, .T. ) ;
#77369=VECTOR ( 'NONE', #35914, 1000.000000000000000 ) ;
#77466=LINE ( 'NONE', #37922, #71551 ) ;
#77467=ORIENTED_EDGE ( 'NONE', *, *, #17895, .T. ) ;
#77546=DIRECTION ( 'NONE',  ( 0.8660254037844380415, -0.5000000000000011102, 0.000000000000000000 ) ) ;
#77575=AXIS2_PLACEMENT_3D ( 'NONE', #71580, #2176, #2678 ) ;
#77595=CARTESIAN_POINT ( 'NONE',  ( -70.00000000000000000, 15.00000000000000000, 59.99999999999999289 ) ) ;
#77600=FACE_OUTER_BOUND ( 'NONE', #68342, .T. ) ;
#77611=DIRECTION ( 'NONE',  ( -1.000000000000000000, -1.156482317317871331E-15, 0.000000000000000000 ) ) ;
#77613=DIRECTION ( 'NONE',  ( -0.8660254037844378194, -0.5000000000000014433, 0.000000000000000000 ) ) ;
#77682=EDGE_CURVE ( 'NONE', #69092, #13291, #82073, .T. ) ;
#77687=ORIENTED_EDGE ( 'NONE', *, *, #69475, .F. ) ;
#77716=VERTEX_POINT ( 'NONE', #66815 ) ;
#77722=CARTESIAN_POINT ( 'NONE',  ( 84.99999999999998579, 14.99999999999999467, -59.99999999999999289 ) ) ;
#77775=ORIENTED_EDGE ( 'NONE', *, *, #88112, .T. ) ;
#77798=EDGE_CURVE ( 'NONE', #27243, #76018, #40888, .T. ) ;
#77834=EDGE_CURVE ( 'NONE', #6810, #57758, #72845, .T. ) ;
#77860=ADVANCED_FACE ( 'NONE', ( #56092 ), #87085, .T. ) ;
#77892=ORIENTED_EDGE ( 'NONE', *, *, #47272, .T. ) ;
#77934=CARTESIAN_POINT ( 'NONE',  ( 18.52134341065868384, 22.64441083166259716, 0.000000000000000000 ) ) ;
#77987=LINE ( 'NONE', #9079, #85450 ) ;
#78012=CARTESIAN_POINT ( 'NONE',  ( -110.0000000000000142, -8.000000000000000000, -9.212605237762117483 ) ) ;
#78040=FACE_OUTER_BOUND ( 'NONE', #26592, .T. ) ;
#78065=DIRECTION ( 'NONE',  ( 0.000000000000000000, 0.000000000000000000, 1.000000000000000000 ) ) ;
#78085=ORIENTED_EDGE ( 'NONE', *, *, #84199, .F. ) ;
#78097=EDGE_CURVE ( 'NONE', #97401, #44408, #45016, .T. ) ;
#78170=EDGE_CURVE ( 'NONE', #60148, #57418, #37785, .T. ) ;
#78213=DIRECTION ( 'NONE',  ( -0.000000000000000000, -0.000000000000000000, -1.000000000000000000 ) ) ;
#78289=ADVANCED_FACE ( 'NONE', ( #54350, #99999, #15356 ), #92908, .T. ) ;
#78333=LINE ( 'NONE', #57003, #30569 ) ;
#78346=EDGE_LOOP ( 'NONE', ( #20288, #15479, #79268, #67613 ) ) ;
#78359=CARTESIAN_POINT ( 'NONE',  ( -110.0000000000000000, 15.00000000000000000, 59.99999999999999289 ) ) ;
#78427=EDGE_CURVE ( 'NONE', #1591, #13682, #18390, .T. ) ;
#78489=EDGE_LOOP ( 'NONE', ( #28511, #76245, #38421, #65586, #21521, #71983, #76323, #53538 ) ) ;
#78537=CARTESIAN_POINT ( 'NONE',  ( -65.00000000000000000, 18.66025403784439973, -54.99999999999999289 ) ) ;
#78579=LINE ( 'NONE', #33465, #42934 ) ;
#78639=CARTESIAN_POINT ( 'NONE',  ( -19.65312891409030271, 93.06504152958497400, 59.99999999999999289 ) ) ;
#78809=EDGE_CURVE ( 'NONE', #48939, #29494, #46691, .T. ) ;
#78881=FACE_OUTER_BOUND ( 'NONE', #90179, .T. ) ;
#78904=ADVANCED_FACE ( 'NONE', ( #7183 ), #91331, .T. ) ;
#78922=AXIS2_PLACEMENT_3D ( 'NONE', #76363, #53530, #13072 ) ;
#78942=DIRECTION ( 'NONE',  ( -0.000000000000000000, 1.000000000000000000, -0.000000000000000000 ) ) ;
#78960=CARTESIAN_POINT ( 'NONE',  ( -13.11024591527734628, 27.99999999999999645, 32.50000000000000000 ) ) ;
#79018=ADVANCED_FACE ( 'NONE', ( #54781 ), #56278, .T. ) ;
#79023=EDGE_LOOP ( 'NONE', ( #98907, #27050, #19163, #27633 ) ) ;
#79093=DIRECTION ( 'NONE',  ( -0.000000000000000000, -0.000000000000000000, -1.000000000000000000 ) ) ;
#79118=DIRECTION ( 'NONE',  ( 0.000000000000000000, 1.000000000000000000, 0.000000000000000000 ) ) ;
#79120=CARTESIAN_POINT ( 'NONE',  ( 110.0000000000000142, 10.00000000000004086, 59.99999999999999289 ) ) ;
#79125=VECTOR ( 'NONE', #46063, 999.9999999999998863 ) ;
#79128=AXIS2_PLACEMENT_3D ( 'NONE', #77595, #76583, #16769 ) ;
#79141=AXIS2_PLACEMENT_3D ( 'NONE', #79120, #16272, #23361 ) ;
#79146=CARTESIAN_POINT ( 'NONE',  ( -110.0000000000000284, 0.000000000000000000, 9.212605237762149457 ) ) ;
#79171=CARTESIAN_POINT ( 'NONE',  ( -110.0000000000000000, 0.000000000000000000, -59.99999999999999289 ) ) ;
#79252=CYLINDRICAL_SURFACE ( 'NONE', #96179, 60.00000000000002132 ) ;
#79263=ORIENTED_EDGE ( 'NONE', *, *, #74236, .F. ) ;
#79268=ORIENTED_EDGE ( 'NONE', *, *, #65026, .T. ) ;
#79271=DIRECTION ( 'NONE',  ( -0.000000000000000000, -0.000000000000000000, -1.000000000000000000 ) ) ;
#79389=CARTESIAN_POINT ( 'NONE',  ( -13.11024591527734451, 6.000000000000000000, -20.00000000000000000 ) ) ;
#79408=DIRECTION ( 'NONE',  ( 1.000000000000000000, 0.000000000000000000, -1.082076799516502204E-16 ) ) ;
#79433=CARTESIAN_POINT ( 'NONE',  ( -110.0000000000000142, 0.000000000000000000, 9.212605237762145904 ) ) ;
#79510=PLANE ( 'NONE',  #40229 ) ;
#79527=VERTEX_POINT ( 'NONE', #62634 ) ;
#79692=VERTEX_POINT ( 'NONE', #75575 ) ;
#79750=VECTOR ( 'NONE', #50057, 1000.000000000000000 ) ;
#79771=LINE ( 'NONE', #10831, #25867 ) ;
#79880=CARTESIAN_POINT ( 'NONE',  ( -70.00000000000000000, 20.00000000000000000, 59.99999999999999289 ) ) ;
#79897=CARTESIAN_POINT ( 'NONE',  ( -55.56624327025929944, 44.99999999999998579, 59.99999999999999289 ) ) ;
#79900=DIRECTION ( 'NONE',  ( 0.000000000000000000, 0.000000000000000000, 1.000000000000000000 ) ) ;
#79915=EDGE_CURVE ( 'NONE', #48468, #39339, #78333, .T. ) ;
#79962=CARTESIAN_POINT ( 'NONE',  ( -13.11024591527734628, 6.000000000000000000, -32.50000000000000000 ) ) ;
#80004=DIRECTION ( 'NONE',  ( 0.5000000000000011102, 0.8660254037844380415, 0.000000000000000000 ) ) ;
#80041=ORIENTED_EDGE ( 'NONE', *, *, #24734, .T. ) ;
#80260=AXIS2_PLACEMENT_3D ( 'NONE', #12112, #81540, #80554 ) ;
#80271=ORIENTED_EDGE ( 'NONE', *, *, #94634, .F. ) ;
#80291=EDGE_CURVE ( 'NONE', #22585, #97093, #72696, .T. ) ;
#80301=ADVANCED_FACE ( 'NONE', ( #63496 ), #93436, .T. ) ;
#80319=DIRECTION ( 'NONE',  ( -1.000000000000000000, 0.000000000000000000, 0.000000000000000000 ) ) ;
#80340=ORIENTED_EDGE ( 'NONE', *, *, #1638, .F. ) ;
#80350=ADVANCED_FACE ( 'NONE', ( #49793 ), #3712, .T. ) ;
#80375=VERTEX_POINT ( 'NONE', #38564 ) ;
#80380=EDGE_CURVE ( 'NONE', #48939, #47538, #60854, .T. ) ;
#80441=CIRCLE ( 'NONE', #88552, 7.500000000000000000 ) ;
#80495=PLANE ( 'NONE',  #25174 ) ;
#80554=DIRECTION ( 'NONE',  ( 0.000000000000000000, -0.000000000000000000, 1.000000000000000000 ) ) ;
#80569=ORIENTED_EDGE ( 'NONE', *, *, #795, .T. ) ;
#80613=PLANE ( 'NONE',  #22631 ) ;
#80615=ADVANCED_FACE ( 'NONE', ( #33482 ), #70470, .T. ) ;
#80677=ADVANCED_FACE ( 'NONE', ( #8678 ), #47165, .T. ) ;
#80691=AXIS2_PLACEMENT_3D ( 'NONE', #23423, #24442, #61429 ) ;
#80727=LINE ( 'NONE', #81216, #36740 ) ;
#80738=VECTOR ( 'NONE', #93040, 1000.000000000000000 ) ;
#80749=AXIS2_PLACEMENT_3D ( 'NONE', #38671, #7781, #68080 ) ;
#80809=CARTESIAN_POINT ( 'NONE',  ( -13.11024591527734628, 27.99999999999999645, 17.00000000000000000 ) ) ;
#80828=ORIENTED_EDGE ( 'NONE', *, *, #91055, .F. ) ;
#80889=EDGE_CURVE ( 'NONE', #7425, #63624, #42924, .T. ) ;
#80894=VECTOR ( 'NONE', #66356, 1000.000000000000114 ) ;
#80926=EDGE_CURVE ( 'NONE', #65117, #33343, #88620, .T. ) ;
#80942=DIRECTION ( 'NONE',  ( 0.8660254037844379305, 0.5000000000000015543, 0.000000000000000000 ) ) ;
#80969=DIRECTION ( 'NONE',  ( 0.000000000000000000, 0.000000000000000000, -1.000000000000000000 ) ) ;
#81044=CARTESIAN_POINT ( 'NONE',  ( -13.11024591527723437, 15.00000000000000000, -25.00000000000017053 ) ) ;
#81216=CARTESIAN_POINT ( 'NONE',  ( -104.9999999999999858, 93.06504152958497400, -54.99999999999999289 ) ) ;
#81251=ORIENTED_EDGE ( 'NONE', *, *, #98036, .T. ) ;
#81384=DIRECTION ( 'NONE',  ( -1.000000000000000000, 0.000000000000000000, 1.082076799516502080E-16 ) ) ;
#81518=ADVANCED_FACE ( 'NONE', ( #53740 ), #38039, .F. ) ;
#81540=DIRECTION ( 'NONE',  ( 0.000000000000000000, 1.000000000000000000, 0.000000000000000000 ) ) ;
#81547=EDGE_CURVE ( 'NONE', #57418, #40435, #20018, .T. ) ;
#81680=CARTESIAN_POINT ( 'NONE',  ( 93.96857342517718337, 10.00000000000001243, -14.21260523776213347 ) ) ;
#81705=CIRCLE ( 'NONE', #21852, 12.50000000000000000 ) ;
#81743=EDGE_LOOP ( 'NONE', ( #42523, #31067, #87415, #57959 ) ) ;
#81754=FACE_OUTER_BOUND ( 'NONE', #78489, .T. ) ;
#81766=ORIENTED_EDGE ( 'NONE', *, *, #99221, .T. ) ;
#81786=DIRECTION ( 'NONE',  ( 1.000000000000000000, 0.000000000000000000, 0.000000000000000000 ) ) ;
#81797=EDGE_CURVE ( 'NONE', #61780, #37352, #33466, .T. ) ;
#81925=DIRECTION ( 'NONE',  ( -0.000000000000000000, 1.000000000000000000, -0.000000000000000000 ) ) ;
#81998=EDGE_CURVE ( 'NONE', #30330, #53652, #100264, .T. ) ;
#82002=ORIENTED_EDGE ( 'NONE', *, *, #44455, .F. ) ;
#82047=EDGE_CURVE ( 'NONE', #49158, #31854, #85605, .T. ) ;
#82073=LINE ( 'NONE', #20236, #77369 ) ;
#82102=ORIENTED_EDGE ( 'NONE', *, *, #91277, .T. ) ;
#82189=VECTOR ( 'NONE', #30735, 1000.000000000000000 ) ;
#82266=PLANE ( 'NONE',  #62570 ) ;
#82272=VERTEX_POINT ( 'NONE', #38758 ) ;
#82359=DIRECTION ( 'NONE',  ( -1.110223024625156343E-15, 1.000000000000000000, 0.000000000000000000 ) ) ;
#82500=DIRECTION ( 'NONE',  ( 1.000000000000000000, 0.000000000000000000, 0.000000000000000000 ) ) ;
#82504=CARTESIAN_POINT ( 'NONE',  ( 49.80235952159635815, 85.00000000000000000, 10.00000000000000000 ) ) ;
#82528=DIRECTION ( 'NONE',  ( -1.000000000000000000, -1.110223024625156343E-15, 0.000000000000000000 ) ) ;
#82546=FACE_OUTER_BOUND ( 'NONE', #68139, .T. ) ;
#82558=ADVANCED_FACE ( 'NONE', ( #78040 ), #61810, .T. ) ;
#82569=ORIENTED_EDGE ( 'NONE', *, *, #95988, .F. ) ;
#82617=CIRCLE ( 'NONE', #27556, 60.00000000000002132 ) ;
#82638=ORIENTED_EDGE ( 'NONE', *, *, #18775, .T. ) ;
#82795=ORIENTED_EDGE ( 'NONE', *, *, #88568, .T. ) ;
#82833=VERTEX_POINT ( 'NONE', #2399 ) ;
#82853=ORIENTED_EDGE ( 'NONE', *, *, #78427, .T. ) ;
#82987=PLANE ( 'NONE',  #78922 ) ;
#83036=DIRECTION ( 'NONE',  ( 0.000000000000000000, 1.000000000000000000, 0.000000000000000000 ) ) ;
#83052=DIRECTION ( 'NONE',  ( -0.000000000000000000, -0.000000000000000000, -1.000000000000000000 ) ) ;
#83098=DIRECTION ( 'NONE',  ( 0.000000000000000000, 0.000000000000000000, 1.000000000000000000 ) ) ;
#83140=AXIS2_PLACEMENT_3D ( 'NONE', #73250, #83363, #81384 ) ;
#83185=CARTESIAN_POINT ( 'NONE',  ( 110.0000000000000000, 0.000000000000000000, -59.99999999999999289 ) ) ;
#83191=DIRECTION ( 'NONE',  ( -0.000000000000000000, -0.000000000000000000, 1.000000000000000000 ) ) ;
#83274=CARTESIAN_POINT ( 'NONE',  ( -13.11024591527723615, 15.00000000000000000, -32.50000000000017053 ) ) ;
#83337=CARTESIAN_POINT ( 'NONE',  ( 79.99999999999998579, 9.999999999999985789, 2.622423327744133559 ) ) ;
#83363=DIRECTION ( 'NONE',  ( -1.082076799516502080E-16, 0.000000000000000000, -1.000000000000000000 ) ) ;
#83384=EDGE_CURVE ( 'NONE', #33261, #9722, #82617, .T. ) ;
#83435=FACE_OUTER_BOUND ( 'NONE', #88718, .T. ) ;
#83443=ORIENTED_EDGE ( 'NONE', *, *, #50687, .F. ) ;
#83473=CARTESIAN_POINT ( 'NONE',  ( -13.11024591527734628, 6.000000000000000000, 25.00000000000000000 ) ) ;
#83581=DIRECTION ( 'NONE',  ( -1.000000000000000000, -0.000000000000000000, -0.000000000000000000 ) ) ;
#83611=ORIENTED_EDGE ( 'NONE', *, *, #23362, .F. ) ;
#83695=DIRECTION ( 'NONE',  ( -1.000000000000000000, 0.000000000000000000, 0.000000000000000000 ) ) ;
#83832=EDGE_CURVE ( 'NONE', #34316, #1591, #49103, .T. ) ;
#83843=ORIENTED_EDGE ( 'NONE', *, *, #31600, .T. ) ;
#83853=ORIENTED_EDGE ( 'NONE', *, *, #76724, .F. ) ;
#83875=EDGE_CURVE ( 'NONE', #76591, #10673, #51841, .T. ) ;
#83894=DIRECTION ( 'NONE',  ( -0.000000000000000000, 1.000000000000000000, -0.000000000000000000 ) ) ;
#83922=CARTESIAN_POINT ( 'NONE',  ( 51.80235952159636525, 85.00000000000000000, 59.99999999999999289 ) ) ;
#83932=AXIS2_PLACEMENT_3D ( 'NONE', #28416, #27923, #4634 ) ;
#83975=VECTOR ( 'NONE', #45213, 1000.000000000000000 ) ;
#83977=AXIS2_PLACEMENT_3D ( 'NONE', #14282, #98406, #90839 ) ;
#84019=ORIENTED_EDGE ( 'NONE', *, *, #88568, .F. ) ;
#84152=CARTESIAN_POINT ( 'NONE',  ( -19.65312891409030271, 9.999999999999994671, -54.99999999999999289 ) ) ;
#84199=EDGE_CURVE ( 'NONE', #26545, #17251, #96997, .T. ) ;
#84278=CARTESIAN_POINT ( 'NONE',  ( -13.11024591527734451, 6.000000000000000000, 45.00000000000000000 ) ) ;
#84289=DIRECTION ( 'NONE',  ( -1.000000000000000000, -1.804112415015878589E-15, 0.000000000000000000 ) ) ;
#84335=CIRCLE ( 'NONE', #14793, 15.50000000000000000 ) ;
#84395=ORIENTED_EDGE ( 'NONE', *, *, #28939, .F. ) ;
#84397=LINE ( 'NONE', #14942, #46406 ) ;
#84432=EDGE_CURVE ( 'NONE', #41822, #91585, #7221, .T. ) ;
#84523=FACE_OUTER_BOUND ( 'NONE', #42458, .T. ) ;
#84660=LINE ( 'NONE', #46100, #35540 ) ;
#84703=DIRECTION ( 'NONE',  ( 0.9746548163034763901, -0.2237140788069380548, 0.000000000000000000 ) ) ;
#84732=DIRECTION ( 'NONE',  ( 0.5000000000000013323, -0.8660254037844378194, 0.000000000000000000 ) ) ;
#84757=CARTESIAN_POINT ( 'NONE',  ( -110.0000000000000142, 4.999999999999999112, -14.21260523776211215 ) ) ;
#84848=EDGE_LOOP ( 'NONE', ( #39179, #496, #60244, #55607, #60003, #82795, #16136, #28396 ) ) ;
#84868=ORIENTED_EDGE ( 'NONE', *, *, #74536, .T. ) ;
#84891=ORIENTED_EDGE ( 'NONE', *, *, #71482, .T. ) ;
#85045=CIRCLE ( 'NONE', #54252, 14.21260523776213347 ) ;
#85107=EDGE_LOOP ( 'NONE', ( #34351, #87969, #63371, #13938, #17688, #56883 ) ) ;
#85218=PLANE ( 'NONE',  #79128 ) ;
#85251=FACE_OUTER_BOUND ( 'NONE', #16854, .T. ) ;
#85256=ORIENTED_EDGE ( 'NONE', *, *, #89789, .T. ) ;
#85335=ORIENTED_EDGE ( 'NONE', *, *, #66078, .T. ) ;
#85336=ORIENTED_EDGE ( 'NONE', *, *, #22702, .T. ) ;
#85350=VECTOR ( 'NONE', #26226, 1000.000000000000000 ) ;
#85362=VECTOR ( 'NONE', #79408, 1000.000000000000000 ) ;
#85390=CARTESIAN_POINT ( 'NONE',  ( -13.11024591527734628, 6.000000000000000000, 32.50000000000000000 ) ) ;
#85417=DIRECTION ( 'NONE',  ( 0.000000000000000000, 0.000000000000000000, 1.000000000000000000 ) ) ;
#85446=DIRECTION ( 'NONE',  ( -1.000000000000000000, -1.804112415015878589E-15, 0.000000000000000000 ) ) ;
#85450=VECTOR ( 'NONE', #39948, 1000.000000000000000 ) ;
#85605=LINE ( 'NONE', #83922, #51699 ) ;
#85697=EDGE_CURVE ( 'NONE', #58741, #50517, #84335, .T. ) ;
#85715=DIRECTION ( 'NONE',  ( -1.000000000000000000, 0.000000000000000000, 0.000000000000000000 ) ) ;
#85730=ORIENTED_EDGE ( 'NONE', *, *, #85697, .T. ) ;
#85770=CARTESIAN_POINT ( 'NONE',  ( 35.39012114306879653, 16.59285393851897084, 10.00000000000000000 ) ) ;
#85880=ORIENTED_EDGE ( 'NONE', *, *, #93770, .T. ) ;
#85967=DIRECTION ( 'NONE',  ( 0.000000000000000000, 1.000000000000000000, 0.000000000000000000 ) ) ;
#85970=DIRECTION ( 'NONE',  ( -1.000000000000000000, -1.387778780781445478E-15, -0.000000000000000000 ) ) ;
#85994=ORIENTED_EDGE ( 'NONE', *, *, #31863, .T. ) ;
#86021=DIRECTION ( 'NONE',  ( 0.000000000000000000, 1.000000000000000000, 0.000000000000000000 ) ) ;
#86046=DIRECTION ( 'NONE',  ( -1.000000000000000000, 0.000000000000000000, 5.984665299743594308E-16 ) ) ;
#86095=AXIS2_PLACEMENT_3D ( 'NONE', #20515, #99010, #22490 ) ;
#86135=AXIS2_PLACEMENT_3D ( 'NONE', #33467, #95324, #25881 ) ;
#86139=CARTESIAN_POINT ( 'NONE',  ( -19.65312891409030271, 93.06504152958497400, -10.00000000000000000 ) ) ;
#86149=AXIS2_PLACEMENT_3D ( 'NONE', #24949, #87832, #17353 ) ;
#86281=CARTESIAN_POINT ( 'NONE',  ( 110.0000000000000000, -8.000000000000000000, 9.212605237762131694 ) ) ;
#86282=DIRECTION ( 'NONE',  ( 1.000000000000000000, 0.000000000000000000, 0.000000000000000000 ) ) ;
#86339=EDGE_CURVE ( 'NONE', #55924, #3243, #52993, .T. ) ;
#86341=AXIS2_PLACEMENT_3D ( 'NONE', #47360, #55445, #85417 ) ;
#86430=VECTOR ( 'NONE', #97280, 1000.000000000000000 ) ;
#86436=FACE_OUTER_BOUND ( 'NONE', #70320, .T. ) ;
#86468=CARTESIAN_POINT ( 'NONE',  ( 39.80235952159635815, 84.99999999999998579, -10.00000000000000000 ) ) ;
#86578=DIRECTION ( 'NONE',  ( -0.5000000000000016653, 0.8660254037844377084, 0.000000000000000000 ) ) ;
#86607=ORIENTED_EDGE ( 'NONE', *, *, #94761, .T. ) ;
#86744=ORIENTED_EDGE ( 'NONE', *, *, #45399, .F. ) ;
#86861=CARTESIAN_POINT ( 'NONE',  ( 105.0000000000000000, 0.000000000000000000, 59.99999999999999289 ) ) ;
#86995=EDGE_CURVE ( 'NONE', #93568, #17251, #11634, .T. ) ;
#87071=ADVANCED_FACE ( 'NONE', ( #47140 ), #32945, .F. ) ;
#87075=AXIS2_PLACEMENT_3D ( 'NONE', #60685, #83052, #29812 ) ;
#87085=PLANE ( 'NONE',  #4621 ) ;
#87102=VECTOR ( 'NONE', #4152, 1000.000000000000000 ) ;
#87118=AXIS2_PLACEMENT_3D ( 'NONE', #50797, #17930, #76125 ) ;
#87128=VERTEX_POINT ( 'NONE', #40031 ) ;
#87160=ORIENTED_EDGE ( 'NONE', *, *, #74227, .F. ) ;
#87383=VERTEX_POINT ( 'NONE', #95059 ) ;
#87415=ORIENTED_EDGE ( 'NONE', *, *, #84199, .T. ) ;
#87466=VERTEX_POINT ( 'NONE', #1321 ) ;
#87508=DIRECTION ( 'NONE',  ( 0.000000000000000000, 0.000000000000000000, -1.000000000000000000 ) ) ;
#87538=DIRECTION ( 'NONE',  ( 1.000000000000000000, 0.000000000000000000, 0.000000000000000000 ) ) ;
#87595=CARTESIAN_POINT ( 'NONE',  ( -65.00000000000000000, 15.00000000000000000, 59.99999999999999289 ) ) ;
#87601=FACE_OUTER_BOUND ( 'NONE', #55118, .T. ) ;
#87726=ORIENTED_EDGE ( 'NONE', *, *, #93833, .F. ) ;
#87768=LINE ( 'NONE', #34486, #32067 ) ;
#87832=DIRECTION ( 'NONE',  ( 0.000000000000000000, -1.000000000000000000, 0.000000000000000000 ) ) ;
#87845=FACE_OUTER_BOUND ( 'NONE', #85107, .T. ) ;
#87969=ORIENTED_EDGE ( 'NONE', *, *, #75424, .T. ) ;
#88000=ADVANCED_FACE ( 'NONE', ( #91937, #68088 ), #36680, .T. ) ;
#88033=ORIENTED_EDGE ( 'NONE', *, *, #73320, .T. ) ;
#88067=EDGE_CURVE ( 'NONE', #87383, #47538, #34260, .T. ) ;
#88086=DIRECTION ( 'NONE',  ( 0.000000000000000000, 0.000000000000000000, -1.000000000000000000 ) ) ;
#88104=ORIENTED_EDGE ( 'NONE', *, *, #6609, .T. ) ;
#88112=EDGE_CURVE ( 'NONE', #98201, #64385, #43783, .T. ) ;
#88121=DIRECTION ( 'NONE',  ( 0.000000000000000000, -1.000000000000000000, 0.000000000000000000 ) ) ;
#88221=CARTESIAN_POINT ( 'NONE',  ( 79.99999999999998579, 20.00000000000000000, -2.622423327744133559 ) ) ;
#88228=VECTOR ( 'NONE', #23275, 1000.000000000000000 ) ;
#88347=ORIENTED_EDGE ( 'NONE', *, *, #7207, .T. ) ;
#88365=EDGE_CURVE ( 'NONE', #5700, #93568, #74611, .T. ) ;
#88441=CARTESIAN_POINT ( 'NONE',  ( -110.0000000000000000, 15.00000000000000000, 59.99999999999999289 ) ) ;
#88552=AXIS2_PLACEMENT_3D ( 'NONE', #98431, #66511, #35612 ) ;
#88555=LINE ( 'NONE', #19121, #53347 ) ;
#88568=EDGE_CURVE ( 'NONE', #51782, #97333, #28863, .T. ) ;
#88620=LINE ( 'NONE', #97195, #33923 ) ;
#88627=CARTESIAN_POINT ( 'NONE',  ( 93.96857342517719758, 15.00000000000000000, 0.000000000000000000 ) ) ;
#88631=AXIS2_PLACEMENT_3D ( 'NONE', #36332, #75360, #4442 ) ;
#88683=EDGE_CURVE ( 'NONE', #36246, #58741, #36947, .T. ) ;
#88695=DIRECTION ( 'NONE',  ( 0.000000000000000000, 0.000000000000000000, -1.000000000000000000 ) ) ;
#88718=EDGE_LOOP ( 'NONE', ( #47667, #65765, #80041, #6054 ) ) ;
#88729=VERTEX_POINT ( 'NONE', #62732 ) ;
#88758=DIRECTION ( 'NONE',  ( -0.000000000000000000, 1.000000000000000000, -0.000000000000000000 ) ) ;
#88760=ORIENTED_EDGE ( 'NONE', *, *, #86995, .T. ) ;
#88781=FACE_BOUND ( 'NONE', #44113, .T. ) ;
#88786=VECTOR ( 'NONE', #49508, 1000.000000000000000 ) ;
#88813=CIRCLE ( 'NONE', #11110, 14.21260523776213347 ) ;
#88832=AXIS2_PLACEMENT_3D ( 'NONE', #17460, #8369, #1780 ) ;
#88853=FACE_OUTER_BOUND ( 'NONE', #43571, .T. ) ;
#88930=VECTOR ( 'NONE', #41223, 1000.000000000000000 ) ;
#88968=PLANE ( 'NONE',  #50608 ) ;
#89041=LINE ( 'NONE', #11489, #32139 ) ;
#89062=EDGE_CURVE ( 'NONE', #16631, #28403, #64760, .T. ) ;
#89094=DIRECTION ( 'NONE',  ( 0.000000000000000000, -0.000000000000000000, 1.000000000000000000 ) ) ;
#89137=DIRECTION ( 'NONE',  ( 0.000000000000000000, 1.000000000000000000, 0.000000000000000000 ) ) ;
#89139=ORIENTED_EDGE ( 'NONE', *, *, #46065, .F. ) ;
#89233=ORIENTED_EDGE ( 'NONE', *, *, #91233, .T. ) ;
#89354=ORIENTED_EDGE ( 'NONE', *, *, #74227, .T. ) ;
#89375=CARTESIAN_POINT ( 'NONE',  ( 110.0000000000000000, 15.00000000000003908, 59.99999999999999289 ) ) ;
#89441=EDGE_CURVE ( 'NONE', #98683, #10673, #76825, .T. ) ;
#89495=DIRECTION ( 'NONE',  ( -0.5000000000000014433, 0.8660254037844379305, 0.000000000000000000 ) ) ;
#89583=DIRECTION ( 'NONE',  ( 0.5000000000000013323, -0.8660254037844378194, 0.000000000000000000 ) ) ;
#89593=CLOSED_SHELL ( 'NONE', ( #96, #3356, #78904, #98140, #48017, #48107, #38625, #3654, #78289, #96993, #73434, #34536, #29475, #27008, #82558, #87071, #47763, #7029, #16556, #66765, #15756, #22075, #35883, #7663, #16428, #51120, #29896, #70757, #36333, #12007, #73204, #59753, #48622, #32100, #21709, #1828, #80350, #35374, #32679, #77860, #43218, #33294, #80301, #80615, #54882, #24472, #57860, #28651, #61823, #51576, #43554, #93386, #51588, #2360, #74579, #72740, #79018, #71888, #39576, #36331, #91931, #64710, #1815, #26844, #66426, #3330, #57332, #80677, #88000, #73721, #32007, #81518 ) ) ;
#89609=CARTESIAN_POINT ( 'NONE',  ( 110.0000000000000000, 0.000000000000000000, 59.99999999999999289 ) ) ;
#89612=VECTOR ( 'NONE', #100019, 1000.000000000000000 ) ;
#89713=CARTESIAN_POINT ( 'NONE',  ( 84.99999999999998579, 15.00000000000000000, 2.106367960268921369 ) ) ;
#89789=EDGE_CURVE ( 'NONE', #22585, #59735, #1420, .T. ) ;
#89889=CYLINDRICAL_SURFACE ( 'NONE', #54323, 7.499999999999992895 ) ;
#89916=CARTESIAN_POINT ( 'NONE',  ( -13.11024591527734628, 27.99999999999999645, 32.50000000000000000 ) ) ;
#89939=AXIS2_PLACEMENT_3D ( 'NONE', #32220, #55013, #87508 ) ;
#89957=DIRECTION ( 'NONE',  ( 0.000000000000000000, -1.000000000000000000, 0.000000000000000000 ) ) ;
#89960=VERTEX_POINT ( 'NONE', #50489 ) ;
#90066=ORIENTED_EDGE ( 'NONE', *, *, #6907, .F. ) ;
#90105=CARTESIAN_POINT ( 'NONE',  ( -13.11024591527723437, 6.000000000000000000, -25.00000000000017053 ) ) ;
#90179=EDGE_LOOP ( 'NONE', ( #96886, #91809, #94687, #66475, #24643, #61359 ) ) ;
#90277=CARTESIAN_POINT ( 'NONE',  ( 93.96857342517719758, 10.00000000000001243, 0.000000000000000000 ) ) ;
#90286=VECTOR ( 'NONE', #21751, 1000.000000000000000 ) ;
#90312=CARTESIAN_POINT ( 'NONE',  ( -55.56624327025929944, 44.99999999999998579, -10.00000000000000000 ) ) ;
#90345=CARTESIAN_POINT ( 'NONE',  ( 39.80235952159635815, 84.99999999999998579, 59.99999999999999289 ) ) ;
#90363=ORIENTED_EDGE ( 'NONE', *, *, #71939, .T. ) ;
#90396=VECTOR ( 'NONE', #66918, 1000.000000000000000 ) ;
#90441=CARTESIAN_POINT ( 'NONE',  ( -57.77801984846012573, 31.16909059156539996, -10.00000000000000178 ) ) ;
#90623=ORIENTED_EDGE ( 'NONE', *, *, #43745, .T. ) ;
#90624=ORIENTED_EDGE ( 'NONE', *, *, #98157, .F. ) ;
#90627=CIRCLE ( 'NONE', #67933, 12.50000000000000000 ) ;
#90647=AXIS2_PLACEMENT_3D ( 'NONE', #31417, #77546, #69915 ) ;
#90752=EDGE_CURVE ( 'NONE', #61436, #6810, #54554, .T. ) ;
#90762=LINE ( 'NONE', #14206, #59406 ) ;
#90839=DIRECTION ( 'NONE',  ( 0.000000000000000000, 0.000000000000000000, 1.000000000000000000 ) ) ;
#90875=ORIENTED_EDGE ( 'NONE', *, *, #3534, .F. ) ;
#90924=VECTOR ( 'NONE', #59471, 1000.000000000000000 ) ;
#91000=CARTESIAN_POINT ( 'NONE',  ( -65.00000000000000000, 18.66025403784439973, 54.99999999999999289 ) ) ;
#91015=CARTESIAN_POINT ( 'NONE',  ( -13.11024591527734628, 6.000000000000000000, -45.00000000000000000 ) ) ;
#91053=ORIENTED_EDGE ( 'NONE', *, *, #86995, .F. ) ;
#91055=EDGE_CURVE ( 'NONE', #18962, #52455, #8959, .T. ) ;
#91086=FACE_OUTER_BOUND ( 'NONE', #27545, .T. ) ;
#91160=EDGE_CURVE ( 'NONE', #17251, #93568, #98280, .T. ) ;
#91225=EDGE_CURVE ( 'NONE', #98683, #58073, #59791, .T. ) ;
#91233=EDGE_CURVE ( 'NONE', #61436, #91371, #90762, .T. ) ;
#91236=CIRCLE ( 'NONE', #15177, 14.21260523776213347 ) ;
#91277=EDGE_CURVE ( 'NONE', #3243, #53003, #45581, .T. ) ;
#91286=LINE ( 'NONE', #68936, #41834 ) ;
#91331=CYLINDRICAL_SURFACE ( 'NONE', #28924, 15.50000000000000000 ) ;
#91371=VERTEX_POINT ( 'NONE', #56174 ) ;
#91378=CARTESIAN_POINT ( 'NONE',  ( 110.0000000000000000, 15.00000000000003908, 59.99999999999999289 ) ) ;
#91414=ORIENTED_EDGE ( 'NONE', *, *, #91613, .F. ) ;
#91426=DIRECTION ( 'NONE',  ( -0.5000000000000013323, 0.8660254037844378194, 0.000000000000000000 ) ) ;
#91430=VERTEX_POINT ( 'NONE', #49587 ) ;
#91513=DIRECTION ( 'NONE',  ( -1.000000000000000000, 0.000000000000000000, 1.082076799516502080E-16 ) ) ;
#91536=CARTESIAN_POINT ( 'NONE',  ( -70.00000000000000000, 15.00000000000000000, -59.99999999999999289 ) ) ;
#91585=VERTEX_POINT ( 'NONE', #93613 ) ;
#91595=DIRECTION ( 'NONE',  ( 1.000000000000000000, 0.000000000000000000, -5.984665299743594308E-16 ) ) ;
#91609=FACE_OUTER_BOUND ( 'NONE', #44178, .T. ) ;
#91613=EDGE_CURVE ( 'NONE', #16870, #27243, #61667, .T. ) ;
#91717=AXIS2_PLACEMENT_3D ( 'NONE', #63022, #47315, #39689 ) ;
#91809=ORIENTED_EDGE ( 'NONE', *, *, #17165, .T. ) ;
#91835=ORIENTED_EDGE ( 'NONE', *, *, #17165, .F. ) ;
#91860=EDGE_CURVE ( 'NONE', #37942, #61780, #23767, .T. ) ;
#91869=VECTOR ( 'NONE', #98469, 1000.000000000000000 ) ;
#91920=CARTESIAN_POINT ( 'NONE',  ( 110.0000000000000000, 15.00000000000003908, 59.99999999999999289 ) ) ;
#91924=DIRECTION ( 'NONE',  ( 0.000000000000000000, 0.000000000000000000, 1.000000000000000000 ) ) ;
#91931=ADVANCED_FACE ( 'NONE', ( #78881 ), #48966, .F. ) ;
#91937=FACE_OUTER_BOUND ( 'NONE', #54378, .T. ) ;
#91975=CARTESIAN_POINT ( 'NONE',  ( 80.66987298107778770, 24.99999999999998579, -10.00000000000000178 ) ) ;
#92097=AXIS2_PLACEMENT_3D ( 'NONE', #65491, #4703, #52278 ) ;
#92138=CARTESIAN_POINT ( 'NONE',  ( -57.04299263576977097, 30.72821847190685673, -10.00000000000000000 ) ) ;
#92535=DIRECTION ( 'NONE',  ( 0.000000000000000000, 0.000000000000000000, 1.000000000000000000 ) ) ;
#92601=CARTESIAN_POINT ( 'NONE',  ( -19.65312891409028850, 79.99999999999991473, 54.99999999999999289 ) ) ;
#92614=DIRECTION ( 'NONE',  ( 0.000000000000000000, 0.000000000000000000, -1.000000000000000000 ) ) ;
#92615=PLANE ( 'NONE',  #98294 ) ;
#92749=CARTESIAN_POINT ( 'NONE',  ( 48.91560817564824504, 80.00000000000000000, -54.99999999999999289 ) ) ;
#92795=DIRECTION ( 'NONE',  ( 5.984665299743594308E-16, 0.000000000000000000, 1.000000000000000000 ) ) ;
#92824=CARTESIAN_POINT ( 'NONE',  ( 66.15274061880275269, 50.14441083166266822, 0.000000000000000000 ) ) ;
#92908=PLANE ( 'NONE',  #80749 ) ;
#92921=LINE ( 'NONE', #46795, #46607 ) ;
#92984=CARTESIAN_POINT ( 'NONE',  ( 105.0000000000000000, 4.999999999999999112, 54.99999999999999289 ) ) ;
#93030=MECHANICAL_DESIGN_GEOMETRIC_PRESENTATION_REPRESENTATION('',(#99461),#68698);
#93040=DIRECTION ( 'NONE',  ( -1.000000000000000000, -0.000000000000000000, -0.000000000000000000 ) ) ;
#93066=DIRECTION ( 'NONE',  ( 0.000000000000000000, 0.000000000000000000, -1.000000000000000000 ) ) ;
#93074=CARTESIAN_POINT ( 'NONE',  ( -86.81108781737714253, 4.999999999999999112, 14.21260523776213347 ) ) ;
#93099=DIRECTION ( 'NONE',  ( 0.000000000000000000, 1.000000000000000000, 0.000000000000000000 ) ) ;
#93119=CARTESIAN_POINT ( 'NONE',  ( 84.99999999999997158, 27.49999999999999645, 59.99999999999999289 ) ) ;
#93181=ORIENTED_EDGE ( 'NONE', *, *, #34434, .T. ) ;
#93233=EDGE_CURVE ( 'NONE', #50517, #58741, #58658, .T. ) ;
#93281=DIRECTION ( 'NONE',  ( 0.000000000000000000, 0.000000000000000000, -1.000000000000000000 ) ) ;
#93318=ORIENTED_EDGE ( 'NONE', *, *, #46570, .T. ) ;
#93386=ADVANCED_FACE ( 'NONE', ( #10531 ), #12029, .T. ) ;
#93436=PLANE ( 'NONE',  #28991 ) ;
#93529=DIRECTION ( 'NONE',  ( 0.8660254037844378194, 0.5000000000000015543, -0.000000000000000000 ) ) ;
#93559=FACE_OUTER_BOUND ( 'NONE', #56629, .T. ) ;
#93561=EDGE_LOOP ( 'NONE', ( #50191, #36191, #58715, #54899 ) ) ;
#93568=VERTEX_POINT ( 'NONE', #16989 ) ;
#93613=CARTESIAN_POINT ( 'NONE',  ( 39.80235952159635815, 84.99999999999998579, -59.99999999999999289 ) ) ;
#93665=VECTOR ( 'NONE', #41663, 1000.000000000000000 ) ;
#93708=CARTESIAN_POINT ( 'NONE',  ( -110.0000000000000142, 10.00000000000000178, 14.21260523776214590 ) ) ;
#93727=VECTOR ( 'NONE', #55416, 1000.000000000000000 ) ;
#93770=EDGE_CURVE ( 'NONE', #43945, #13446, #18345, .T. ) ;
#93833=EDGE_CURVE ( 'NONE', #49158, #33261, #2063, .T. ) ;
#93963=DIRECTION ( 'NONE',  ( -1.000000000000000000, 0.000000000000000000, 0.000000000000000000 ) ) ;
#93964=CARTESIAN_POINT ( 'NONE',  ( -13.11024591527734628, 0.000000000000000000, -32.50000000000000000 ) ) ;
#93984=LINE ( 'NONE', #10860, #93727 ) ;
#94029=CARTESIAN_POINT ( 'NONE',  ( 110.0000000000000000, 15.00000000000003908, 59.99999999999999289 ) ) ;
#94095=CARTESIAN_POINT ( 'NONE',  ( -13.11024591527723615, 27.99999999999999645, -32.50000000000017053 ) ) ;
#94130=PLANE ( 'NONE',  #67426 ) ;
#94279=DIRECTION ( 'NONE',  ( 1.000000000000000000, 1.804112415015878984E-15, 0.000000000000000000 ) ) ;
#94289=CARTESIAN_POINT ( 'NONE',  ( 51.80235952159636525, 85.00000000000000000, 59.99999999999999289 ) ) ;
#94433=DIRECTION ( 'NONE',  ( -1.000000000000000000, 0.000000000000000000, 0.000000000000000000 ) ) ;
#94434=VERTEX_POINT ( 'NONE', #28228 ) ;
#94437=VECTOR ( 'NONE', #5808, 1000.000000000000000 ) ;
#94528=CARTESIAN_POINT ( 'NONE',  ( 38.90713653809340400, 79.99999999999998579, 54.99999999999999289 ) ) ;
#94599=ORIENTED_EDGE ( 'NONE', *, *, #88683, .F. ) ;
#94634=EDGE_CURVE ( 'NONE', #9722, #61780, #12429, .T. ) ;
#94664=DIRECTION ( 'NONE',  ( 0.000000000000000000, 0.000000000000000000, -1.000000000000000000 ) ) ;
#94666=EDGE_LOOP ( 'NONE', ( #15036, #15835 ) ) ;
#94687=ORIENTED_EDGE ( 'NONE', *, *, #98036, .F. ) ;
#94761=EDGE_CURVE ( 'NONE', #28403, #44016, #32600, .T. ) ;
#94840=DIRECTION ( 'NONE',  ( 0.000000000000000000, 0.000000000000000000, 1.000000000000000000 ) ) ;
#94967=CARTESIAN_POINT ( 'NONE',  ( -70.00000000000000000, 15.00000000000000000, -59.99999999999999289 ) ) ;
#94999=VECTOR ( 'NONE', #96853, 1000.000000000000000 ) ;
#95059=CARTESIAN_POINT ( 'NONE',  ( 65.48286763772492236, 61.30466486950707150, 0.000000000000000000 ) ) ;
#95077=ORIENTED_EDGE ( 'NONE', *, *, #306, .T. ) ;
#95170=CARTESIAN_POINT ( 'NONE',  ( 110.0000000000000142, 20.00000000000000000, 1.387778780781445676E-14 ) ) ;
#95180=EDGE_LOOP ( 'NONE', ( #57562, #16943 ) ) ;
#95214=CARTESIAN_POINT ( 'NONE',  ( -19.65312891409030271, 93.06504152958497400, -10.00000000000000000 ) ) ;
#95238=FACE_OUTER_BOUND ( 'NONE', #31497, .T. ) ;
#95279=AXIS2_PLACEMENT_3D ( 'NONE', #14508, #39271, #92535 ) ;
#95309=ORIENTED_EDGE ( 'NONE', *, *, #69508, .F. ) ;
#95324=DIRECTION ( 'NONE',  ( -0.000000000000000000, -1.000000000000000000, -0.000000000000000000 ) ) ;
#95326=ORIENTED_EDGE ( 'NONE', *, *, #61740, .T. ) ;
#95460=ORIENTED_EDGE ( 'NONE', *, *, #32045, .T. ) ;
#95620=FACE_OUTER_BOUND ( 'NONE', #38817, .T. ) ;
#95743=CARTESIAN_POINT ( 'NONE',  ( 110.0000000000000000, -8.000000000000000000, -9.212605237762131694 ) ) ;
#95817=CARTESIAN_POINT ( 'NONE',  ( -55.56624327025929944, 44.99999999999998579, 10.00000000000000000 ) ) ;
#95837=CARTESIAN_POINT ( 'NONE',  ( 105.0000000000000000, 4.999999999999999112, 59.99999999999999289 ) ) ;
#95881=LINE ( 'NONE', #20335, #64328 ) ;
#95958=CARTESIAN_POINT ( 'NONE',  ( 79.99999999999990052, 93.06504152958508769, -54.99999999999999289 ) ) ;
#95959=ORIENTED_EDGE ( 'NONE', *, *, #23362, .T. ) ;
#95988=EDGE_CURVE ( 'NONE', #33601, #40913, #35445, .T. ) ;
#96026=CARTESIAN_POINT ( 'NONE',  ( -13.11024591527734628, 6.000000000000000000, 20.00000000000000000 ) ) ;
#96037=DIRECTION ( 'NONE',  ( -1.000000000000000000, 0.000000000000000000, 1.082076799516502204E-16 ) ) ;
#96137=CARTESIAN_POINT ( 'NONE',  ( -70.00000000000000000, 20.00000000000000000, -59.99999999999999289 ) ) ;
#96179=AXIS2_PLACEMENT_3D ( 'NONE', #2723, #78213, #71623 ) ;
#96189=CARTESIAN_POINT ( 'NONE',  ( 105.0000000000000000, -8.000000000000000000, -14.21260523776213347 ) ) ;
#96320=DIRECTION ( 'NONE',  ( 0.000000000000000000, 0.000000000000000000, -1.000000000000000000 ) ) ;
#96339=DIRECTION ( 'NONE',  ( 5.984665299743594308E-16, 0.000000000000000000, 1.000000000000000000 ) ) ;
#96374=VECTOR ( 'NONE', #44054, 1000.000000000000000 ) ;
#96455=FACE_OUTER_BOUND ( 'NONE', #27388, .T. ) ;
#96496=ORIENTED_EDGE ( 'NONE', *, *, #37610, .F. ) ;
#96499=VECTOR ( 'NONE', #89495, 999.9999999999998863 ) ;
#96576=ORIENTED_EDGE ( 'NONE', *, *, #28789, .T. ) ;
#96586=CARTESIAN_POINT ( 'NONE',  ( 105.0000000000000000, 4.999999999999999112, 14.21260523776213347 ) ) ;
#96639=CARTESIAN_POINT ( 'NONE',  ( -19.65312891409030271, 5.000000000000004441, -54.99999999999999289 ) ) ;
#96852=CARTESIAN_POINT ( 'NONE',  ( -70.00000000000000000, 20.00000000000000000, -59.99999999999999289 ) ) ;
#96853=DIRECTION ( 'NONE',  ( 1.000000000000000000, 1.804112415015878984E-15, -1.082076799516502204E-16 ) ) ;
#96861=PLANE ( 'NONE',  #56445 ) ;
#96886=ORIENTED_EDGE ( 'NONE', *, *, #98732, .T. ) ;
#96913=AXIS2_PLACEMENT_3D ( 'NONE', #57968, #42748, #80319 ) ;
#96937=AXIS2_PLACEMENT_3D ( 'NONE', #39168, #70082, #695 ) ;
#96993=ADVANCED_FACE ( 'NONE', ( #47289 ), #79252, .F. ) ;
#96997=LINE ( 'NONE', #80809, #71226 ) ;
#96998=CARTESIAN_POINT ( 'NONE',  ( -105.0000000000000000, 0.000000000000000000, 59.99999999999999289 ) ) ;
#97009=VECTOR ( 'NONE', #46020, 1000.000000000000000 ) ;
#97023=DIRECTION ( 'NONE',  ( -0.000000000000000000, -1.000000000000000000, -0.000000000000000000 ) ) ;
#97047=DIRECTION ( 'NONE',  ( -0.000000000000000000, 1.000000000000000000, -0.000000000000000000 ) ) ;
#97093=VERTEX_POINT ( 'NONE', #16152 ) ;
#97107=EDGE_LOOP ( 'NONE', ( #63868, #99305, #42091, #63349 ) ) ;
#97115=DIRECTION ( 'NONE',  ( -0.000000000000000000, 1.000000000000000000, -0.000000000000000000 ) ) ;
#97172=CARTESIAN_POINT ( 'NONE',  ( 66.15274061880275269, 50.14441083166266822, 0.000000000000000000 ) ) ;
#97195=CARTESIAN_POINT ( 'NONE',  ( 93.96857342517718337, -8.000000000000000000, -9.212605237762131694 ) ) ;
#97280=DIRECTION ( 'NONE',  ( 0.000000000000000000, 0.000000000000000000, -1.000000000000000000 ) ) ;
#97321=CARTESIAN_POINT ( 'NONE',  ( -86.81108781737714253, -8.000000000000000000, -9.212605237762131694 ) ) ;
#97322=ORIENTED_EDGE ( 'NONE', *, *, #57818, .T. ) ;
#97333=VERTEX_POINT ( 'NONE', #74381 ) ;
#97358=CARTESIAN_POINT ( 'NONE',  ( 93.96857342517718337, 0.000000000000000000, 9.212605237762133470 ) ) ;
#97401=VERTEX_POINT ( 'NONE', #37328 ) ;
#97406=ORIENTED_EDGE ( 'NONE', *, *, #1496, .T. ) ;
#97422=PLANE ( 'NONE',  #48422 ) ;
#97437=DIRECTION ( 'NONE',  ( 0.5000000000000014433, -0.8660254037844379305, 0.000000000000000000 ) ) ;
#97522=VECTOR ( 'NONE', #97893, 1000.000000000000000 ) ;
#97587=EDGE_CURVE ( 'NONE', #9722, #8604, #33230, .T. ) ;
#97617=CARTESIAN_POINT ( 'NONE',  ( 110.0000000000000000, 0.000000000000000000, 59.99999999999999289 ) ) ;
#97640=DIRECTION ( 'NONE',  ( -1.000000000000000000, 0.000000000000000000, 5.984665299743594308E-16 ) ) ;
#97689=ORIENTED_EDGE ( 'NONE', *, *, #38257, .T. ) ;
#97763=ORIENTED_EDGE ( 'NONE', *, *, #35519, .T. ) ;
#97764=CARTESIAN_POINT ( 'NONE',  ( -110.0000000000000000, 15.00000000000000000, 59.99999999999999289 ) ) ;
#97802=ORIENTED_EDGE ( 'NONE', *, *, #22702, .F. ) ;
#97824=LINE ( 'NONE', #34995, #94999 ) ;
#97893=DIRECTION ( 'NONE',  ( -0.000000000000000000, 1.000000000000000000, -0.000000000000000000 ) ) ;
#97945=VECTOR ( 'NONE', #42195, 1000.000000000000000 ) ;
#98036=EDGE_CURVE ( 'NONE', #77716, #77081, #5595, .T. ) ;
#98084=ORIENTED_EDGE ( 'NONE', *, *, #59559, .F. ) ;
#98095=CARTESIAN_POINT ( 'NONE',  ( -13.11024591527734628, 6.000000000000000000, 32.50000000000000000 ) ) ;
#98110=LINE ( 'NONE', #52982, #15716 ) ;
#98140=ADVANCED_FACE ( 'NONE', ( #35608 ), #74129, .T. ) ;
#98157=EDGE_CURVE ( 'NONE', #17199, #21265, #72466, .T. ) ;
#98165=VECTOR ( 'NONE', #15650, 1000.000000000000000 ) ;
#98201=VERTEX_POINT ( 'NONE', #2042 ) ;
#98226=CARTESIAN_POINT ( 'NONE',  ( 38.90713653809340400, 79.99999999999998579, 10.00000000000000000 ) ) ;
#98258=DIRECTION ( 'NONE',  ( -1.000000000000000000, 0.000000000000000000, 0.000000000000000000 ) ) ;
#98265=CARTESIAN_POINT ( 'NONE',  ( -13.11024591527734451, 27.99999999999999645, 48.00000000000000000 ) ) ;
#98280=CIRCLE ( 'NONE', #25438, 15.50000000000000000 ) ;
#98294=AXIS2_PLACEMENT_3D ( 'NONE', #30276, #93099, #30784 ) ;
#98295=CARTESIAN_POINT ( 'NONE',  ( 75.48286763772496499, 43.98415679381830756, 1.224646799147354045E-15 ) ) ;
#98328=ORIENTED_EDGE ( 'NONE', *, *, #55295, .T. ) ;
#98406=DIRECTION ( 'NONE',  ( 0.000000000000000000, 1.000000000000000000, 0.000000000000000000 ) ) ;
#98417=EDGE_LOOP ( 'NONE', ( #41817, #141, #35948, #97322 ) ) ;
#98431=CARTESIAN_POINT ( 'NONE',  ( -13.11024591527734628, 27.99999999999999645, 32.50000000000000000 ) ) ;
#98469=DIRECTION ( 'NONE',  ( -0.000000000000000000, -0.000000000000000000, -1.000000000000000000 ) ) ;
#98683=VERTEX_POINT ( 'NONE', #60585 ) ;
#98732=EDGE_CURVE ( 'NONE', #94434, #13291, #18893, .T. ) ;
#98779=VERTEX_POINT ( 'NONE', #60826 ) ;
#98783=AXIS2_PLACEMENT_3D ( 'NONE', #55670, #71414, #2516 ) ;
#98872=EDGE_CURVE ( 'NONE', #36590, #24906, #59332, .T. ) ;
#98901=CARTESIAN_POINT ( 'NONE',  ( -13.11024591527723615, 27.99999999999999645, -32.50000000000017053 ) ) ;
#98907=ORIENTED_EDGE ( 'NONE', *, *, #10886, .F. ) ;
#98935=DIRECTION ( 'NONE',  ( 0.8575671445351807920, -0.5143720371616018472, 0.000000000000000000 ) ) ;
#99010=DIRECTION ( 'NONE',  ( 0.000000000000000000, -1.000000000000000000, 0.000000000000000000 ) ) ;
#99138=ORIENTED_EDGE ( 'NONE', *, *, #26184, .F. ) ;
#99221=EDGE_CURVE ( 'NONE', #39339, #60148, #71645, .T. ) ;
#99241=EDGE_CURVE ( 'NONE', #91430, #87128, #81705, .T. ) ;
#99247=VECTOR ( 'NONE', #34203, 1000.000000000000000 ) ;
#99305=ORIENTED_EDGE ( 'NONE', *, *, #12211, .T. ) ;
#99461=STYLED_ITEM('',(#100310),#46005);
#99517=FACE_BOUND ( 'NONE', #95180, .T. ) ;
#99619=CARTESIAN_POINT ( 'NONE',  ( 110.0000000000000000, 15.00000000000003908, -59.99999999999999289 ) ) ;
#99717=CIRCLE ( 'NONE', #55928, 60.00000000000002132 ) ;
#99816=ORIENTED_EDGE ( 'NONE', *, *, #80926, .F. ) ;
#99825=CARTESIAN_POINT ( 'NONE',  ( -13.11024591527734628, 6.000000000000000000, -32.50000000000000000 ) ) ;
#99852=AXIS2_PLACEMENT_3D ( 'NONE', #34988, #4096, #25923 ) ;
#99882=ORIENTED_EDGE ( 'NONE', *, *, #16457, .F. ) ;
#99987=AXIS2_PLACEMENT_3D ( 'NONE', #89916, #5284, #11899 ) ;
#99999=FACE_OUTER_BOUND ( 'NONE', #11821, .T. ) ;
#100019=DIRECTION ( 'NONE',  ( -1.000000000000000000, -1.804112415015878984E-15, 1.082076799516502204E-16 ) ) ;
#100033=ORIENTED_EDGE ( 'NONE', *, *, #91277, .F. ) ;
#100044=EDGE_CURVE ( 'NONE', #55924, #82833, #29213, .T. ) ;
#100097=CARTESIAN_POINT ( 'NONE',  ( 110.0000000000000000, 15.00000000000000000, -9.212605237762131694 ) ) ;
#100116=DIRECTION ( 'NONE',  ( 0.000000000000000000, 0.000000000000000000, -1.000000000000000000 ) ) ;
#100133=VECTOR ( 'NONE', #86282, 1000.000000000000000 ) ;
#100230=CARTESIAN_POINT ( 'NONE',  ( -86.81108781737714253, -8.000000000000000000, 14.21260523776213347 ) ) ;
#100264=LINE ( 'NONE', #47535, #97009 ) ;
#100265=DIRECTION ( 'NONE',  ( 0.000000000000000000, 0.000000000000000000, -1.000000000000000000 ) ) ;
#100284=LINE ( 'NONE', #61753, #98165 ) ;
#100286=VERTEX_POINT ( 'NONE', #90441 ) ;
#100304=COLOUR_RGB('Dark Blue',0.08,0.2,0.34);
#100305=FILL_AREA_STYLE_COLOUR('',#100304);
#100306=FILL_AREA_STYLE('',(#100305));
#100307=SURFACE_STYLE_FILL_AREA(#100306);
#100308=SURFACE_SIDE_STYLE('',(#100307));
#100309=SURFACE_STYLE_USAGE(.BOTH.,#100308);
#100310=PRESENTATION_STYLE_ASSIGNMENT((#100309));
ENDSEC;
END-ISO-10303-21;
